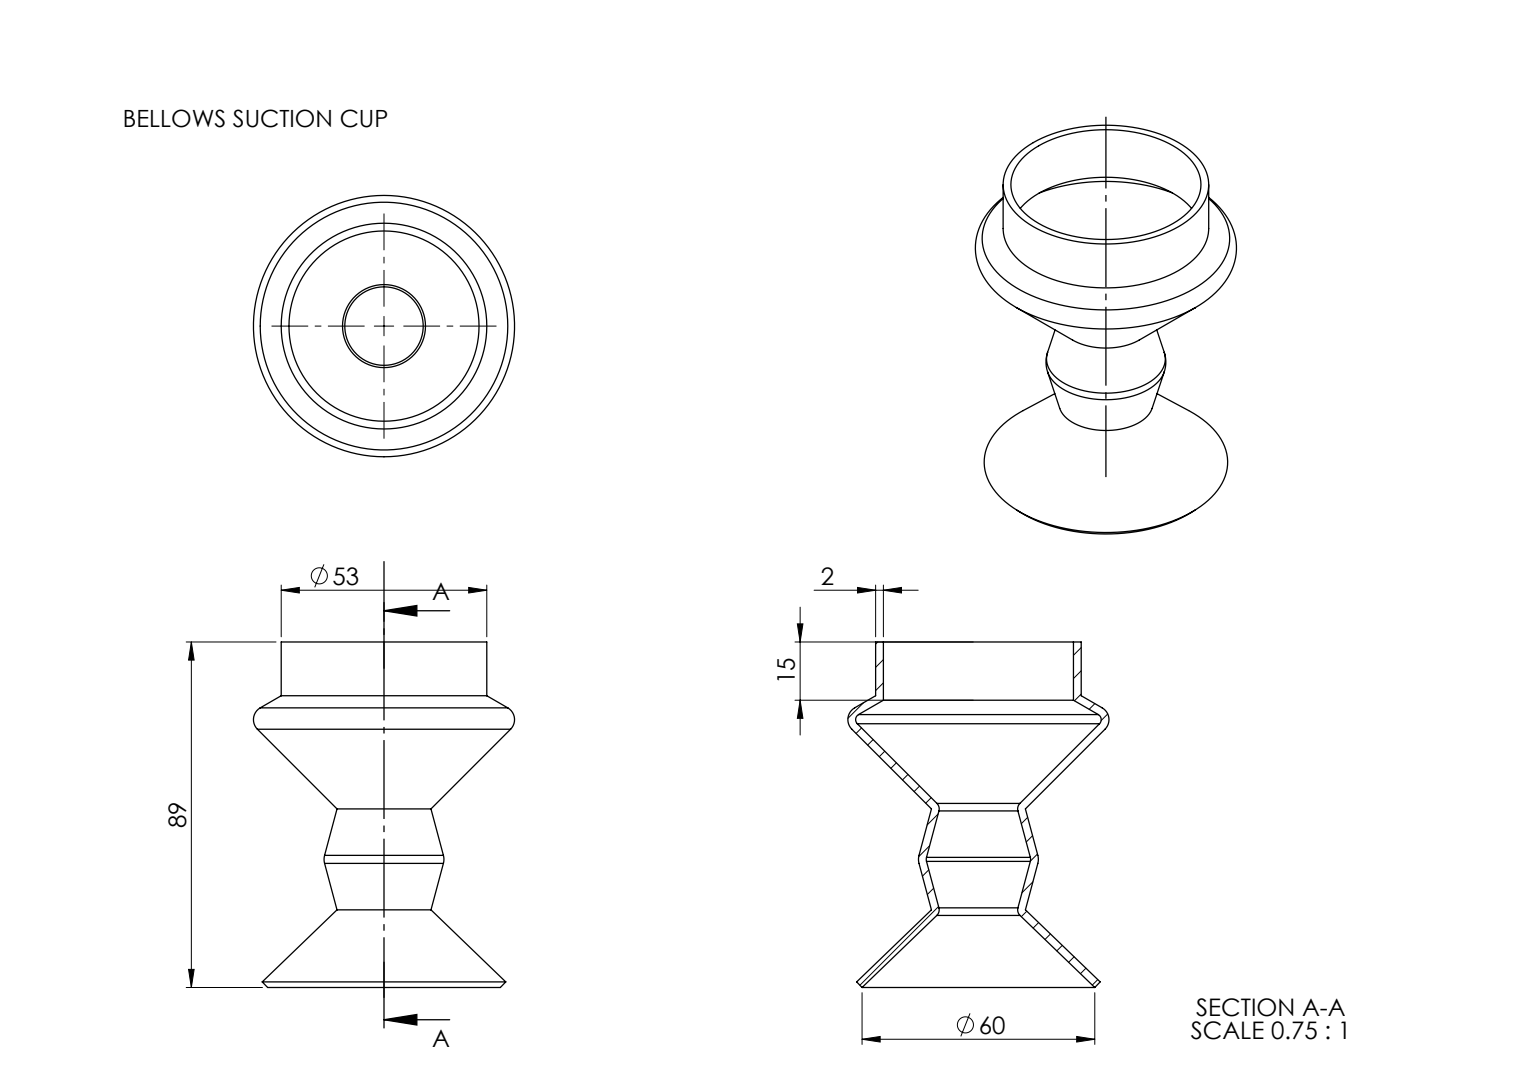
ISO-10303-21;
HEADER;
FILE_DESCRIPTION (('STEP AP214'),
    '1' );
FILE_NAME ('bellows suction cup.step',
    '2026-10-02T18:08:48',
    ( '' ),
    ( '' ),
    'SwSTEP 2.0',
    'SolidWorks 2026',
    '' );
FILE_SCHEMA (( 'AUTOMOTIVE_DESIGN' ));
ENDSEC;

DATA;
#110=CARTESIAN_POINT ( 'NONE',  ( 2.757615341152813402E-15, -45.51763809020504681, 0.000000000000000000 ) ) ;
#122=CARTESIAN_POINT ( 'NONE',  ( 0.000000000000000000, -21.99999999999999645, 0.000000000000000000 ) ) ;
#136=CIRCLE ( 'NONE', #19335, 15.31593959127081384 ) ;
#143=DIRECTION ( 'NONE',  ( -1.224646799147353454E-16, 1.000000000000000000, -0.000000000000000000 ) ) ;
#174=EDGE_LOOP ( 'NONE', ( #26748, #4103, #22808, #13833 ) ) ;
#178=CARTESIAN_POINT ( 'NONE',  ( 31.22091420962414787, -23.06066017177981209, 3.823459265327032686E-15 ) ) ;
#199=ORIENTED_EDGE ( 'NONE', *, *, #10938, .T. ) ;
#210=CLOSED_SHELL ( 'NONE', ( #8729, #14117, #31790, #11042, #12512, #8597, #17021, #15792, #28040, #1353, #2874, #26985, #12292, #25228, #17408, #25082, #11130, #24622, #12986, #14394, #9494, #16184, #21021, #7313, #8316, #7903, #7462, #29778, #24071, #10707, #8891, #2660, #1384, #1595, #31267, #2291, #15122, #887, #228, #13989, #650, #29273, #23959 ) ) ;
#213=CIRCLE ( 'NONE', #1854, 31.22091420962414787 ) ;
#215=DIRECTION ( 'NONE',  ( 1.224646799147353454E-16, -1.000000000000000000, 0.000000000000000000 ) ) ;
#228=ADVANCED_FACE ( 'NONE', ( #2232 ), #22152, .F. ) ;
#229=DIRECTION ( 'NONE',  ( 0.7202789989107551971, -0.6936844842780615084, 0.000000000000000000 ) ) ;
#231=( GEOMETRIC_REPRESENTATION_CONTEXT ( 3 ) GLOBAL_UNCERTAINTY_ASSIGNED_CONTEXT ( ( #25969 ) ) GLOBAL_UNIT_ASSIGNED_CONTEXT ( ( #31394, #13204, #25908 ) ) REPRESENTATION_CONTEXT ( 'NONE', 'WORKASPACE' ) );
#237=AXIS2_PLACEMENT_3D ( 'NONE', #10911, #18810, #13315 ) ;
#253=LINE ( 'NONE', #21716, #27788 ) ;
#265=DIRECTION ( 'NONE',  ( 1.224646799147353454E-16, -1.000000000000000000, 0.000000000000000000 ) ) ;
#266=ORIENTED_EDGE ( 'NONE', *, *, #7688, .T. ) ;
#281=FACE_OUTER_BOUND ( 'NONE', #10068, .T. ) ;
#284=DIRECTION ( 'NONE',  ( -1.224646799147353454E-16, 1.000000000000000000, -0.000000000000000000 ) ) ;
#374=CIRCLE ( 'NONE', #19015, 10.72870458603808075 ) ;
#401=CONICAL_SURFACE ( 'NONE', #22876, 24.50000000000000000, 0.7853981633974463916 ) ;
#429=CIRCLE ( 'NONE', #33304, 4.000000000000014211 ) ;
#464=DIRECTION ( 'NONE',  ( -1.000000000000000000, 0.000000000000000000, 0.000000000000000000 ) ) ;
#474=ORIENTED_EDGE ( 'NONE', *, *, #17841, .F. ) ;
#555=FACE_OUTER_BOUND ( 'NONE', #3316, .T. ) ;
#628=DIRECTION ( 'NONE',  ( -1.224646799147353454E-16, 1.000000000000000000, -0.000000000000000000 ) ) ;
#650=ADVANCED_FACE ( 'NONE', ( #26598 ), #1853, .T. ) ;
#676=AXIS2_PLACEMENT_3D ( 'NONE', #19715, #30162, #1674 ) ;
#706=CARTESIAN_POINT ( 'NONE',  ( 2.757615341152813402E-15, -45.51763809020504681, 0.000000000000000000 ) ) ;
#708=DIRECTION ( 'NONE',  ( 0.000000000000000000, -0.000000000000000000, -1.000000000000000000 ) ) ;
#869=APPLICATION_CONTEXT ( 'automotive_design' ) ;
#887=ADVANCED_FACE ( 'NONE', ( #25022 ), #29271, .F. ) ;
#958=DIRECTION ( 'NONE',  ( -1.000000000000000000, 0.000000000000000000, 0.000000000000000000 ) ) ;
#1000=DIRECTION ( 'NONE',  ( -1.224646799147353454E-16, 1.000000000000000000, -0.000000000000000000 ) ) ;
#1009=EDGE_LOOP ( 'NONE', ( #6385, #19811, #24661, #9041 ) ) ;
#1026=CARTESIAN_POINT ( 'NONE',  ( -8.761981113183991350E-16, -15.84529946162075298, 0.000000000000000000 ) ) ;
#1032=ORIENTED_EDGE ( 'NONE', *, *, #9068, .F. ) ;
#1054=ORIENTED_EDGE ( 'NONE', *, *, #1897, .T. ) ;
#1063=EDGE_CURVE ( 'NONE', #21883, #11212, #23262, .T. ) ;
#1088=VERTEX_POINT ( 'NONE', #12842 ) ;
#1136=AXIS2_PLACEMENT_3D ( 'NONE', #18668, #12050, #13680 ) ;
#1137=CIRCLE ( 'NONE', #17065, 10.11000150615022264 ) ;
#1163=DIRECTION ( 'NONE',  ( 0.2588190451025240146, -0.9659258262890673130, 0.000000000000000000 ) ) ;
#1165=FACE_OUTER_BOUND ( 'NONE', #17941, .T. ) ;
#1195=DIRECTION ( 'NONE',  ( -1.000000000000000000, 0.000000000000000000, 0.000000000000000000 ) ) ;
#1257=ORIENTED_EDGE ( 'NONE', *, *, #27744, .T. ) ;
#1353=ADVANCED_FACE ( 'NONE', ( #14831 ), #15022, .F. ) ;
#1355=DIRECTION ( 'NONE',  ( -1.000000000000000000, -1.309225264888156377E-16, 0.000000000000000000 ) ) ;
#1376=AXIS2_PLACEMENT_3D ( 'NONE', #6186, #27460, #21818 ) ;
#1384=ADVANCED_FACE ( 'NONE', ( #23749 ), #5887, .F. ) ;
#1388=VECTOR ( 'NONE', #20093, 999.9999999999998863 ) ;
#1443=DIRECTION ( 'NONE',  ( -1.224646799147353454E-16, 1.000000000000000000, -0.000000000000000000 ) ) ;
#1465=AXIS2_PLACEMENT_3D ( 'NONE', #20580, #4942, #2371 ) ;
#1503=DIRECTION ( 'NONE',  ( -1.224646799147353454E-16, 1.000000000000000000, -0.000000000000000000 ) ) ;
#1561=EDGE_LOOP ( 'NONE', ( #16202, #13374, #12638, #10013 ) ) ;
#1595=ADVANCED_FACE ( 'NONE', ( #555 ), #27605, .F. ) ;
#1608=DIRECTION ( 'NONE',  ( -1.224646799147353454E-16, 1.000000000000000000, -0.000000000000000000 ) ) ;
#1612=CARTESIAN_POINT ( 'NONE',  ( -10.11000150615021909, -45.00000000000000000, 0.000000000000000000 ) ) ;
#1674=DIRECTION ( 'NONE',  ( -1.000000000000000000, -1.416100796715761110E-16, 0.000000000000000000 ) ) ;
#1707=CIRCLE ( 'NONE', #20926, 10.18398033115917656 ) ;
#1766=CARTESIAN_POINT ( 'NONE',  ( 2.757615341152813402E-15, -45.51763809020504681, 0.000000000000000000 ) ) ;
#1770=AXIS2_PLACEMENT_3D ( 'NONE', #2717, #20916, #25712 ) ;
#1797=AXIS2_PLACEMENT_3D ( 'NONE', #2551, #23660, #26230 ) ;
#1853=TOROIDAL_SURFACE ( 'NONE', #7348, 12.11607355459420177, 2.000000000000000000 ) ;
#1854=AXIS2_PLACEMENT_3D ( 'NONE', #13967, #24431, #32646 ) ;
#1864=CARTESIAN_POINT ( 'NONE',  ( 13.38432950954957512, -58.51673569255127205, 1.639107629260334588E-15 ) ) ;
#1886=ORIENTED_EDGE ( 'NONE', *, *, #20671, .F. ) ;
#1897=EDGE_CURVE ( 'NONE', #21971, #4339, #29772, .T. ) ;
#1957=ORIENTED_EDGE ( 'NONE', *, *, #17449, .T. ) ;
#1981=FACE_OUTER_BOUND ( 'NONE', #8042, .T. ) ;
#1996=ORIENTED_EDGE ( 'NONE', *, *, #9547, .T. ) ;
#2013=TOROIDAL_SURFACE ( 'NONE', #21222, 12.11607355459420177, 2.000000000000000000 ) ;
#2034=DIRECTION ( 'NONE',  ( -1.224646799147353454E-16, 1.000000000000000000, -0.000000000000000000 ) ) ;
#2232=FACE_OUTER_BOUND ( 'NONE', #1009, .T. ) ;
#2254=VERTEX_POINT ( 'NONE', #178 ) ;
#2262=FACE_OUTER_BOUND ( 'NONE', #5128, .T. ) ;
#2265=TOROIDAL_SURFACE ( 'NONE', #29108, 12.11607355459420177, 2.000000000000000000 ) ;
#2291=ADVANCED_FACE ( 'NONE', ( #13746 ), #401, .F. ) ;
#2357=CIRCLE ( 'NONE', #6728, 12.11607355459420354 ) ;
#2367=FACE_OUTER_BOUND ( 'NONE', #33613, .T. ) ;
#2371=DIRECTION ( 'NONE',  ( -1.000000000000000000, 0.000000000000000000, 0.000000000000000000 ) ) ;
#2379=EDGE_CURVE ( 'NONE', #7355, #7743, #13581, .T. ) ;
#2383=AXIS2_PLACEMENT_3D ( 'NONE', #26930, #10991, #16152 ) ;
#2387=ORIENTED_EDGE ( 'NONE', *, *, #22718, .T. ) ;
#2402=SURFACE_SIDE_STYLE ('',( #5653 ) ) ;
#2408=AXIS2_PLACEMENT_3D ( 'NONE', #21011, #215, #25978 ) ;
#2453=DIRECTION ( 'NONE',  ( 0.2588190451025257355, -0.9659258262890668689, 0.000000000000000000 ) ) ;
#2480=COLOUR_RGB ( '', 0.66274510, 0.83137255, 0.94901961) ;
#2481=EDGE_LOOP ( 'NONE', ( #22705, #4855, #29179, #20689 ) ) ;
#2551=CARTESIAN_POINT ( 'NONE',  ( 2.694222958124179176E-15, -45.00000000000001421, 0.000000000000000000 ) ) ;
#2593=CARTESIAN_POINT ( 'NONE',  ( 11.45223628611453215, -57.99999999999999289, 1.402494451086933009E-15 ) ) ;
#2601=AXIS2_PLACEMENT_3D ( 'NONE', #3611, #27453, #1355 ) ;
#2660=ADVANCED_FACE ( 'NONE', ( #12691, #12522 ), #4281, .F. ) ;
#2690=ORIENTED_EDGE ( 'NONE', *, *, #25523, .T. ) ;
#2717=CARTESIAN_POINT ( 'NONE',  ( -2.815509657234710744E-16, -20.70096189432334555, 0.000000000000000000 ) ) ;
#2720=FACE_OUTER_BOUND ( 'NONE', #7788, .T. ) ;
#2729=EDGE_LOOP ( 'NONE', ( #11660, #5888, #17586, #12988 ) ) ;
#2789=CARTESIAN_POINT ( 'NONE',  ( 30.00000000000001066, -91.00000000000000000, 0.000000000000000000 ) ) ;
#2856=CARTESIAN_POINT ( 'NONE',  ( 24.50000000000000000, -16.99999999999999289, 3.000384657911015469E-15 ) ) ;
#2874=ADVANCED_FACE ( 'NONE', ( #5478 ), #31637, .T. ) ;
#2898=ORIENTED_EDGE ( 'NONE', *, *, #20671, .T. ) ;
#2940=EDGE_LOOP ( 'NONE', ( #4959, #14793, #18981, #27682 ) ) ;
#2949=DIRECTION ( 'NONE',  ( 0.000000000000000000, -0.000000000000000000, -1.000000000000000000 ) ) ;
#3047=DIRECTION ( 'NONE',  ( -0.7071067811865462405, 0.7071067811865489050, 0.000000000000000000 ) ) ;
#3083=CARTESIAN_POINT ( 'NONE',  ( 5.204170427930421283E-15, -70.99969134886156041, 0.000000000000000000 ) ) ;
#3143=AXIS2_PLACEMENT_3D ( 'NONE', #16484, #26940, #3440 ) ;
#3150=DIRECTION ( 'NONE',  ( -1.000000000000000000, -1.416100796715761110E-16, 0.000000000000000000 ) ) ;
#3165=AXIS2_PLACEMENT_3D ( 'NONE', #16128, #3242, #24176 ) ;
#3191=AXIS2_PLACEMENT_3D ( 'NONE', #22795, #4600, #25545 ) ;
#3242=DIRECTION ( 'NONE',  ( -1.224646799147353454E-16, 1.000000000000000000, -0.000000000000000000 ) ) ;
#3289=EDGE_CURVE ( 'NONE', #15868, #29257, #7629, .T. ) ;
#3316=EDGE_LOOP ( 'NONE', ( #474, #19189, #20666, #19232 ) ) ;
#3375=VECTOR ( 'NONE', #16248, 1000.000000000000114 ) ;
#3422=EDGE_CURVE ( 'NONE', #4339, #20029, #29557, .T. ) ;
#3440=DIRECTION ( 'NONE',  ( 1.000000000000000000, 0.000000000000000000, 1.224646799147352714E-16 ) ) ;
#3450=DIRECTION ( 'NONE',  ( 1.224646799147353454E-16, -1.000000000000000000, 0.000000000000000000 ) ) ;
#3455=AXIS2_PLACEMENT_3D ( 'NONE', #29112, #7846, #8183 ) ;
#3465=DIRECTION ( 'NONE',  ( -1.000000000000000000, 0.000000000000000000, 0.000000000000000000 ) ) ;
#3487=ORIENTED_EDGE ( 'NONE', *, *, #23060, .T. ) ;
#3554=LINE ( 'NONE', #11609, #25895 ) ;
#3565=ORIENTED_EDGE ( 'NONE', *, *, #25296, .F. ) ;
#3608=AXIS2_PLACEMENT_3D ( 'NONE', #1026, #24229, #21987 ) ;
#3611=CARTESIAN_POINT ( 'NONE',  ( -8.761981113183991350E-16, -15.84529946162075298, 0.000000000000000000 ) ) ;
#3664=DIRECTION ( 'NONE',  ( 1.000000000000000000, 0.000000000000000000, 1.224646799147353947E-16 ) ) ;
#3707=EDGE_CURVE ( 'NONE', #11212, #14916, #27280, .T. ) ;
#3757=EDGE_CURVE ( 'NONE', #16950, #4399, #21280, .T. ) ;
#3768=DIRECTION ( 'NONE',  ( -0.2588190451025255689, -0.9659258262890669799, 3.169619151431825338E-17 ) ) ;
#3773=CARTESIAN_POINT ( 'NONE',  ( 3.469446951953614189E-15, -45.00000000000000000, 0.000000000000000000 ) ) ;
#3890=FILL_AREA_STYLE_COLOUR ( '', #2480 ) ;
#3963=CARTESIAN_POINT ( 'NONE',  ( 4.412827539393359662E-15, -59.03347138510255832, 0.000000000000000000 ) ) ;
#3970=AXIS2_PLACEMENT_3D ( 'NONE', #27710, #1443, #17589 ) ;
#3977=VERTEX_POINT ( 'NONE', #10259 ) ;
#4088=DIRECTION ( 'NONE',  ( 1.000000000000000000, 0.000000000000000000, 0.000000000000000000 ) ) ;
#4103=ORIENTED_EDGE ( 'NONE', *, *, #8318, .T. ) ;
#4130=ORIENTED_EDGE ( 'NONE', *, *, #27703, .T. ) ;
#4144=VECTOR ( 'NONE', #9708, 1000.000000000000114 ) ;
#4169=DIRECTION ( 'NONE',  ( -0.2588190451025238481, -0.9659258262890674240, 3.169619151431803768E-17 ) ) ;
#4196=FACE_OUTER_BOUND ( 'NONE', #4510, .T. ) ;
#4221=DIRECTION ( 'NONE',  ( -1.224646799147353454E-16, 1.000000000000000000, -0.000000000000000000 ) ) ;
#4244=CARTESIAN_POINT ( 'NONE',  ( 6.054684311146244891E-15, -72.44024934668307480, 0.000000000000000000 ) ) ;
#4276=ORIENTED_EDGE ( 'NONE', *, *, #9547, .F. ) ;
#4281=PLANE ( 'NONE',  #6435 ) ;
#4315=ORIENTED_EDGE ( 'NONE', *, *, #7894, .F. ) ;
#4339=VERTEX_POINT ( 'NONE', #20056 ) ;
#4356=ORIENTED_EDGE ( 'NONE', *, *, #7565, .T. ) ;
#4373=DIRECTION ( 'NONE',  ( -1.000000000000000000, 0.000000000000000000, 0.000000000000000000 ) ) ;
#4386=APPLICATION_CONTEXT ( 'automotive_design' ) ;
#4399=VERTEX_POINT ( 'NONE', #27772 ) ;
#4418=EDGE_CURVE ( 'NONE', #7411, #6369, #6462, .T. ) ;
#4430=LINE ( 'NONE', #17313, #13313 ) ;
#4507=CARTESIAN_POINT ( 'NONE',  ( -13.38432950954956624, -58.51673569255127205, 0.000000000000000000 ) ) ;
#4508=CARTESIAN_POINT ( 'NONE',  ( 15.31642273298461632, -59.03347138510255832, 1.875720807433735970E-15 ) ) ;
#4510=EDGE_LOOP ( 'NONE', ( #15697, #18450, #22380, #31090 ) ) ;
#4526=EDGE_CURVE ( 'NONE', #11830, #7617, #7016, .T. ) ;
#4531=CIRCLE ( 'NONE', #1770, 30.91025403784432868 ) ;
#4534=ORIENTED_EDGE ( 'NONE', *, *, #1063, .T. ) ;
#4536=CIRCLE ( 'NONE', #10037, 24.49999999999999645 ) ;
#4539=CARTESIAN_POINT ( 'NONE',  ( 2.521031746877078694E-15, -43.58578643762690064, 0.000000000000000000 ) ) ;
#4600=DIRECTION ( 'NONE',  ( -1.224646799147353454E-16, 1.000000000000000000, -0.000000000000000000 ) ) ;
#4602=DIRECTION ( 'NONE',  ( -1.000000000000000000, 0.000000000000000000, 0.000000000000000000 ) ) ;
#4609=EDGE_CURVE ( 'NONE', #7355, #27495, #33250, .T. ) ;
#4623=CARTESIAN_POINT ( 'NONE',  ( -26.50000000000000355, -2.000000000000000000, 0.000000000000000000 ) ) ;
#4635=CARTESIAN_POINT ( 'NONE',  ( 32.63512777199724724, -24.47487373415290790, 3.996650476574133167E-15 ) ) ;
#4665=ORIENTED_EDGE ( 'NONE', *, *, #3422, .T. ) ;
#4679=DIRECTION ( 'NONE',  ( -1.000000000000000000, -1.224646799147353454E-16, 0.000000000000000000 ) ) ;
#4682=ORIENTED_EDGE ( 'NONE', *, *, #29841, .T. ) ;
#4708=CARTESIAN_POINT ( 'NONE',  ( 7.428728520588063561E-18, -23.06066017177981564, 0.000000000000000000 ) ) ;
#4855=ORIENTED_EDGE ( 'NONE', *, *, #12029, .T. ) ;
#4915=ORIENTED_EDGE ( 'NONE', *, *, #8318, .F. ) ;
#4931=SHAPE_DEFINITION_REPRESENTATION ( #13749, #19696 ) ;
#4942=DIRECTION ( 'NONE',  ( -1.224646799147353454E-16, 1.000000000000000000, -0.000000000000000000 ) ) ;
#4952=PRODUCT ( 'bellows suction cup', 'bellows suction cup', '', ( #23473 ) ) ;
#4959=ORIENTED_EDGE ( 'NONE', *, *, #27703, .F. ) ;
#5000=ORIENTED_EDGE ( 'NONE', *, *, #11667, .F. ) ;
#5007=DIRECTION ( 'NONE',  ( -1.224646799147353207E-16, -1.499759782661857882E-32, 1.000000000000000000 ) ) ;
#5021=FACE_OUTER_BOUND ( 'NONE', #24340, .T. ) ;
#5042=EDGE_CURVE ( 'NONE', #28529, #17976, #11406, .T. ) ;
#5044=CARTESIAN_POINT ( 'NONE',  ( -29.99999999999999645, -91.00000000000000000, 3.673940397442059967E-15 ) ) ;
#5128=EDGE_LOOP ( 'NONE', ( #30565, #20332, #24416, #11247 ) ) ;
#5131=ORIENTED_EDGE ( 'NONE', *, *, #16178, .T. ) ;
#5143=PRESENTATION_STYLE_ASSIGNMENT (( #12870 ) ) ;
#5178=EDGE_CURVE ( 'NONE', #6369, #7411, #5928, .T. ) ;
#5187=DIRECTION ( 'NONE',  ( -0.8660254037844369313, -0.5000000000000028866, 1.060575238724904943E-16 ) ) ;
#5201=AXIS2_PLACEMENT_3D ( 'NONE', #9756, #9587, #15086 ) ;
#5259=EDGE_LOOP ( 'NONE', ( #28388, #30221, #18020, #27449 ) ) ;
#5271=DIRECTION ( 'NONE',  ( -1.224646799147353454E-16, 1.000000000000000000, -0.000000000000000000 ) ) ;
#5285=DIRECTION ( 'NONE',  ( -0.6936844842780661713, 0.7202789989107508672, 0.000000000000000000 ) ) ;
#5286=EDGE_CURVE ( 'NONE', #20029, #1088, #429, .T. ) ;
#5312=DIRECTION ( 'NONE',  ( 0.2583678462756400229, 0.9660466117175129375, 3.164093559440580996E-17 ) ) ;
#5385=VERTEX_POINT ( 'NONE', #27561 ) ;
#5430=CARTESIAN_POINT ( 'NONE',  ( 3.469446951953614189E-15, -45.00000000000000000, 0.000000000000000000 ) ) ;
#5478=FACE_OUTER_BOUND ( 'NONE', #19566, .T. ) ;
#5559=ORIENTED_EDGE ( 'NONE', *, *, #9068, .T. ) ;
#5582=CIRCLE ( 'NONE', #9960, 26.50000000000000000 ) ;
#5597=ORIENTED_EDGE ( 'NONE', *, *, #11873, .T. ) ;
#5600=EDGE_CURVE ( 'NONE', #7743, #23590, #21725, .T. ) ;
#5645=ORIENTED_EDGE ( 'NONE', *, *, #12029, .F. ) ;
#5653=SURFACE_STYLE_FILL_AREA ( #29319 ) ;
#5672=AXIS2_PLACEMENT_3D ( 'NONE', #23110, #23461, #33923 ) ;
#5817=CIRCLE ( 'NONE', #7458, 10.17814985357208890 ) ;
#5830=CARTESIAN_POINT ( 'NONE',  ( 5.204170427930421283E-15, -70.99969134886156041, 0.000000000000000000 ) ) ;
#5838=DIRECTION ( 'NONE',  ( -0.7202789989107549751, -0.6936844842780617304, 8.820873705091161919E-17 ) ) ;
#5887=CYLINDRICAL_SURFACE ( 'NONE', #33662, 24.49999999999999645 ) ;
#5888=ORIENTED_EDGE ( 'NONE', *, *, #24657, .F. ) ;
#5900=EDGE_CURVE ( 'NONE', #1088, #9464, #33248, .T. ) ;
#5928=CIRCLE ( 'NONE', #25094, 13.38432950954957157 ) ;
#6007=ORIENTED_EDGE ( 'NONE', *, *, #23213, .T. ) ;
#6141=DIRECTION ( 'NONE',  ( 1.224646799147353454E-16, -1.000000000000000000, 0.000000000000000000 ) ) ;
#6169=AXIS2_PLACEMENT_3D ( 'NONE', #11647, #32574, #17149 ) ;
#6186=CARTESIAN_POINT ( 'NONE',  ( 0.000000000000000000, 0.000000000000000000, 0.000000000000000000 ) ) ;
#6190=AXIS2_PLACEMENT_3D ( 'NONE', #32901, #9400, #19883 ) ;
#6220=AXIS2_PLACEMENT_3D ( 'NONE', #24367, #19056, #14067 ) ;
#6224=VERTEX_POINT ( 'NONE', #5044 ) ;
#6245=AXIS2_PLACEMENT_3D ( 'NONE', #6662, #25544, #4088 ) ;
#6275=EDGE_CURVE ( 'NONE', #29257, #31380, #12941, .T. ) ;
#6312=MECHANICAL_DESIGN_GEOMETRIC_PRESENTATION_REPRESENTATION('',(#28758),#28244);
#6336=CARTESIAN_POINT ( 'NONE',  ( 10.18398033115918189, -70.48295565631028126, 1.443142760386851780E-15 ) ) ;
#6346=CARTESIAN_POINT ( 'NONE',  ( -10.11607355459419644, -70.99969134886156041, 0.000000000000000000 ) ) ;
#6369=VERTEX_POINT ( 'NONE', #18613 ) ;
#6380=EDGE_CURVE ( 'NONE', #7743, #14916, #15865, .T. ) ;
#6385=ORIENTED_EDGE ( 'NONE', *, *, #30392, .F. ) ;
#6393=CARTESIAN_POINT ( 'NONE',  ( 24.49999999999999645, -22.99999999999999645, 3.000384657911015074E-15 ) ) ;
#6398=CIRCLE ( 'NONE', #1465, 30.00000000000000711 ) ;
#6407=DIRECTION ( 'NONE',  ( -1.224646799147353207E-16, -1.499759782661857882E-32, 1.000000000000000000 ) ) ;
#6409=VECTOR ( 'NONE', #31627, 1000.000000000000000 ) ;
#6435=AXIS2_PLACEMENT_3D ( 'NONE', #4623, #25733, #12862 ) ;
#6437=DIRECTION ( 'NONE',  ( -1.000000000000000000, -1.224646799147353454E-16, 0.000000000000000000 ) ) ;
#6462=CIRCLE ( 'NONE', #9190, 13.38432950954957157 ) ;
#6574=CARTESIAN_POINT ( 'NONE',  ( -7.347880794884122694E-16, -16.99999999999999645, 0.000000000000000000 ) ) ;
#6593=CARTESIAN_POINT ( 'NONE',  ( 4.159479030958464888E-15, -56.96472381958990638, 0.000000000000000000 ) ) ;
#6600=EDGE_LOOP ( 'NONE', ( #30266, #4130, #15362, #12431 ) ) ;
#6662=CARTESIAN_POINT ( 'NONE',  ( 2.757615341152813402E-15, -45.51763809020504681, 0.000000000000000000 ) ) ;
#6696=FACE_OUTER_BOUND ( 'NONE', #2729, .T. ) ;
#6701=ORIENTED_EDGE ( 'NONE', *, *, #5600, .F. ) ;
#6724=LINE ( 'NONE', #6393, #23733 ) ;
#6728=AXIS2_PLACEMENT_3D ( 'NONE', #22944, #25686, #7146 ) ;
#6756=AXIS2_PLACEMENT_3D ( 'NONE', #122, #10614, #20758 ) ;
#6780=AXIS2_PLACEMENT_3D ( 'NONE', #33203, #30630, #9706 ) ;
#6845=EDGE_CURVE ( 'NONE', #28463, #33921, #21228, .T. ) ;
#6849=CARTESIAN_POINT ( 'NONE',  ( 24.49999999999999289, -1.999999999999995337, 3.000384657911015074E-15 ) ) ;
#6866=LINE ( 'NONE', #30885, #1388 ) ;
#6869=ORIENTED_EDGE ( 'NONE', *, *, #32222, .T. ) ;
#6905=VECTOR ( 'NONE', #3047, 999.9999999999998863 ) ;
#6909=CARTESIAN_POINT ( 'NONE',  ( -10.17814985357208535, -45.51763809020504681, 1.246463863941915894E-15 ) ) ;
#6976=VERTEX_POINT ( 'NONE', #6346 ) ;
#7016=CIRCLE ( 'NONE', #3191, 24.49999999999999645 ) ;
#7146=DIRECTION ( 'NONE',  ( -1.000000000000000000, 0.000000000000000000, 0.000000000000000000 ) ) ;
#7258=EDGE_CURVE ( 'NONE', #25648, #9464, #13557, .T. ) ;
#7279=DIRECTION ( 'NONE',  ( -1.000000000000000000, -1.111257322145974683E-16, 0.000000000000000000 ) ) ;
#7289=CYLINDRICAL_SURFACE ( 'NONE', #27068, 26.50000000000000000 ) ;
#7313=ADVANCED_FACE ( 'NONE', ( #20595 ), #22849, .T. ) ;
#7348=AXIS2_PLACEMENT_3D ( 'NONE', #5830, #16309, #26765 ) ;
#7355=VERTEX_POINT ( 'NONE', #27790 ) ;
#7381=FACE_OUTER_BOUND ( 'NONE', #10798, .T. ) ;
#7411=VERTEX_POINT ( 'NONE', #1864 ) ;
#7457=VERTEX_POINT ( 'NONE', #2856 ) ;
#7458=AXIS2_PLACEMENT_3D ( 'NONE', #706, #11192, #20998 ) ;
#7462=ADVANCED_FACE ( 'NONE', ( #22811 ), #20355, .T. ) ;
#7519=AXIS2_PLACEMENT_3D ( 'NONE', #3773, #19565, #27281 ) ;
#7533=EDGE_LOOP ( 'NONE', ( #12921, #21559, #5131, #12948 ) ) ;
#7565=EDGE_CURVE ( 'NONE', #33921, #28463, #1137, .T. ) ;
#7581=TOROIDAL_SURFACE ( 'NONE', #28853, 30.16025403784430736, 3.500000000000010658 ) ;
#7617=VERTEX_POINT ( 'NONE', #6849 ) ;
#7629=LINE ( 'NONE', #8297, #24513 ) ;
#7677=CARTESIAN_POINT ( 'NONE',  ( 6.054684311146244891E-15, -72.44024934668307480, 0.000000000000000000 ) ) ;
#7680=DIRECTION ( 'NONE',  ( -1.000000000000000000, 0.000000000000000000, 0.000000000000000000 ) ) ;
#7688=EDGE_CURVE ( 'NONE', #23106, #2254, #12165, .T. ) ;
#7689=FACE_OUTER_BOUND ( 'NONE', #32083, .T. ) ;
#7743=VERTEX_POINT ( 'NONE', #24459 ) ;
#7751=DIRECTION ( 'NONE',  ( -1.000000000000000000, -1.224646799147353454E-16, 0.000000000000000000 ) ) ;
#7752=AXIS2_PLACEMENT_3D ( 'NONE', #17729, #25954, #33327 ) ;
#7780=AXIS2_PLACEMENT_3D ( 'NONE', #25350, #12307, #15584 ) ;
#7788=EDGE_LOOP ( 'NONE', ( #3565, #9159, #26412, #199 ) ) ;
#7822=CIRCLE ( 'NONE', #16072, 31.22091420962414787 ) ;
#7838=TOROIDAL_SURFACE ( 'NONE', #27017, 12.11000150615021553, 1.999999999999992228 ) ;
#7846=DIRECTION ( 'NONE',  ( -1.224646799147353454E-16, 1.000000000000000000, -0.000000000000000000 ) ) ;
#7849=DIRECTION ( 'NONE',  ( -1.000000000000000000, 0.000000000000000000, 0.000000000000000000 ) ) ;
#7857=CARTESIAN_POINT ( 'NONE',  ( -31.22091420962414787, -23.06066017177981919, 0.000000000000000000 ) ) ;
#7894=EDGE_CURVE ( 'NONE', #18620, #6224, #31838, .T. ) ;
#7903=ADVANCED_FACE ( 'NONE', ( #4196 ), #14881, .T. ) ;
#7922=CARTESIAN_POINT ( 'NONE',  ( 12.11000150615021909, -45.00000000000000000, 1.483047458217648827E-15 ) ) ;
#7935=CARTESIAN_POINT ( 'NONE',  ( 0.000000000000000000, -21.99999999999999645, 0.000000000000000000 ) ) ;
#7998=AXIS2_PLACEMENT_3D ( 'NONE', #32435, #29863, #16842 ) ;
#8001=ORIENTED_EDGE ( 'NONE', *, *, #22244, .F. ) ;
#8021=CARTESIAN_POINT ( 'NONE',  ( 5.814984965855610735E-15, -70.48295565631028126, 0.000000000000000000 ) ) ;
#8042=EDGE_LOOP ( 'NONE', ( #4534, #24009, #8001, #1886 ) ) ;
#8079=AXIS2_PLACEMENT_3D ( 'NONE', #16861, #27321, #20637 ) ;
#8131=VECTOR ( 'NONE', #23794, 1000.000000000000000 ) ;
#8156=DIRECTION ( 'NONE',  ( 0.2583678462756386907, 0.9660466117175132705, 3.164093559440564356E-17 ) ) ;
#8183=DIRECTION ( 'NONE',  ( -1.000000000000000000, -1.087251435804610394E-16, 0.000000000000000000 ) ) ;
#8195=DIRECTION ( 'NONE',  ( -1.224646799147353454E-16, 1.000000000000000000, -0.000000000000000000 ) ) ;
#8255=PRODUCT_DEFINITION ( 'UNKNOWN', '', #14809, #19552 ) ;
#8286=CONICAL_SURFACE ( 'NONE', #25293, 10.72870458603808075, 0.8042044335707554392 ) ;
#8297=CARTESIAN_POINT ( 'NONE',  ( 10.72870458603808608, -72.44024934668307480, 0.000000000000000000 ) ) ;
#8316=ADVANCED_FACE ( 'NONE', ( #18370 ), #12678, .T. ) ;
#8318=EDGE_CURVE ( 'NONE', #29257, #6224, #20927, .T. ) ;
#8324=EDGE_CURVE ( 'NONE', #21971, #25648, #20608, .T. ) ;
#8358=CARTESIAN_POINT ( 'NONE',  ( 4.222871413987100692E-15, -57.48236190979495319, 0.000000000000000000 ) ) ;
#8370=ORIENTED_EDGE ( 'NONE', *, *, #14830, .T. ) ;
#8372=ORIENTED_EDGE ( 'NONE', *, *, #11319, .F. ) ;
#8597=ADVANCED_FACE ( 'NONE', ( #26587 ), #8286, .F. ) ;
#8631=DIRECTION ( 'NONE',  ( -1.000000000000000000, 0.000000000000000000, 0.000000000000000000 ) ) ;
#8682=DIRECTION ( 'NONE',  ( -1.000000000000000000, -1.063101997391471025E-16, 0.000000000000000000 ) ) ;
#8729=ADVANCED_FACE ( 'NONE', ( #16626 ), #2265, .T. ) ;
#8737=CARTESIAN_POINT ( 'NONE',  ( -10.17814985357208535, -45.51763809020504681, 0.000000000000000000 ) ) ;
#8845=CIRCLE ( 'NONE', #25292, 10.11607355459420177 ) ;
#8891=ADVANCED_FACE ( 'NONE', ( #11797 ), #27418, .T. ) ;
#8908=CONICAL_SURFACE ( 'NONE', #33581, 30.00000000000000711, 0.7665918932241471140 ) ;
#8911=CIRCLE ( 'NONE', #13317, 1.999999999999993117 ) ;
#8938=CONICAL_SURFACE ( 'NONE', #17725, 32.63512777199724724, 0.7853981633974471688 ) ;
#8990=CARTESIAN_POINT ( 'NONE',  ( 32.63512777199724724, -24.47487373415290790, 3.996650476574133167E-15 ) ) ;
#9041=ORIENTED_EDGE ( 'NONE', *, *, #30437, .T. ) ;
#9068=EDGE_CURVE ( 'NONE', #12231, #28463, #11073, .T. ) ;
#9071=DIRECTION ( 'NONE',  ( -1.224646799147353454E-16, 1.000000000000000000, -0.000000000000000000 ) ) ;
#9080=EDGE_CURVE ( 'NONE', #23590, #27495, #5582, .T. ) ;
#9086=CIRCLE ( 'NONE', #28279, 2.000000000000013767 ) ;
#9124=ORIENTED_EDGE ( 'NONE', *, *, #27744, .F. ) ;
#9159=ORIENTED_EDGE ( 'NONE', *, *, #27274, .F. ) ;
#9190=AXIS2_PLACEMENT_3D ( 'NONE', #30500, #25023, #27431 ) ;
#9344=DIRECTION ( 'NONE',  ( -1.224646799147353454E-16, 1.000000000000000000, -0.000000000000000000 ) ) ;
#9372=CIRCLE ( 'NONE', #25834, 31.38736896855613523 ) ;
#9400=DIRECTION ( 'NONE',  ( -1.224646799147353454E-16, 1.000000000000000000, -0.000000000000000000 ) ) ;
#9441=CONICAL_SURFACE ( 'NONE', #6169, 13.38432950954957157, 0.2613323016132363952 ) ;
#9464=VERTEX_POINT ( 'NONE', #28228 ) ;
#9466=DIRECTION ( 'NONE',  ( -1.000000000000000000, 0.000000000000000000, 0.000000000000000000 ) ) ;
#9483=ORIENTED_EDGE ( 'NONE', *, *, #5286, .F. ) ;
#9494=ADVANCED_FACE ( 'NONE', ( #25994 ), #25855, .T. ) ;
#9523=FACE_OUTER_BOUND ( 'NONE', #26108, .T. ) ;
#9540=STYLED_ITEM ( 'NONE', ( #5143 ), #15260 ) ;
#9547=EDGE_CURVE ( 'NONE', #12231, #23106, #14342, .T. ) ;
#9587=DIRECTION ( 'NONE',  ( -1.224646799147353454E-16, 1.000000000000000000, -0.000000000000000000 ) ) ;
#9593=AXIS2_PLACEMENT_3D ( 'NONE', #17629, #20555, #28090 ) ;
#9594=DIRECTION ( 'NONE',  ( 0.7071067811865460184, 0.7071067811865489050, 8.659560562354914369E-17 ) ) ;
#9643=DIRECTION ( 'NONE',  ( -1.000000000000000000, -1.239088197126291063E-16, 0.000000000000000000 ) ) ;
#9706=DIRECTION ( 'NONE',  ( -1.000000000000000000, -1.309225264888156377E-16, 0.000000000000000000 ) ) ;
#9708=DIRECTION ( 'NONE',  ( 0.7202789989107551971, -0.6936844842780615084, 0.000000000000000000 ) ) ;
#9756=CARTESIAN_POINT ( 'NONE',  ( -2.571758278209442450E-15, -1.999999999999998224, 0.000000000000000000 ) ) ;
#9829=DIRECTION ( 'NONE',  ( -0.2583678462756388572, 0.9660466117175131595, 0.000000000000000000 ) ) ;
#9865=DIRECTION ( 'NONE',  ( -1.000000000000000000, -1.224646799147353454E-16, 0.000000000000000000 ) ) ;
#9960=AXIS2_PLACEMENT_3D ( 'NONE', #12482, #5271, #17988 ) ;
#10013=ORIENTED_EDGE ( 'NONE', *, *, #13215, .T. ) ;
#10035=ORIENTED_EDGE ( 'NONE', *, *, #32348, .T. ) ;
#10037=AXIS2_PLACEMENT_3D ( 'NONE', #26116, #18239, #20294 ) ;
#10068=EDGE_LOOP ( 'NONE', ( #18616, #17669, #31630, #5559 ) ) ;
#10093=DIRECTION ( 'NONE',  ( -1.224646799147353454E-16, 1.000000000000000000, -0.000000000000000000 ) ) ;
#10117=ORIENTED_EDGE ( 'NONE', *, *, #11873, .F. ) ;
#10135=DIRECTION ( 'NONE',  ( -1.224646799147353454E-16, 1.000000000000000000, -0.000000000000000000 ) ) ;
#10212=VECTOR ( 'NONE', #9829, 1000.000000000000114 ) ;
#10259=CARTESIAN_POINT ( 'NONE',  ( 10.11607355459420710, -70.99969134886156041, 1.238861709857297692E-15 ) ) ;
#10291=ORIENTED_EDGE ( 'NONE', *, *, #33593, .T. ) ;
#10316=DIRECTION ( 'NONE',  ( 1.000000000000000000, 0.000000000000000000, 1.224646799147353700E-16 ) ) ;
#10340=CARTESIAN_POINT ( 'NONE',  ( -30.16025403784430736, -22.00000000000000000, 0.000000000000000000 ) ) ;
#10372=ORIENTED_EDGE ( 'NONE', *, *, #22463, .T. ) ;
#10411=EDGE_LOOP ( 'NONE', ( #23839, #23627, #18896, #13145 ) ) ;
#10431=DIRECTION ( 'NONE',  ( -1.224646799147353454E-16, 1.000000000000000000, -0.000000000000000000 ) ) ;
#10573=CIRCLE ( 'NONE', #33001, 2.000000000000000000 ) ;
#10583=ORIENTED_EDGE ( 'NONE', *, *, #25296, .T. ) ;
#10601=CARTESIAN_POINT ( 'NONE',  ( -24.49999999999999645, -17.00000000000000000, 0.000000000000000000 ) ) ;
#10607=DIRECTION ( 'NONE',  ( -1.224646799147353454E-16, 1.000000000000000000, -0.000000000000000000 ) ) ;
#10614=DIRECTION ( 'NONE',  ( -1.224646799147353454E-16, 1.000000000000000000, -0.000000000000000000 ) ) ;
#10625=EDGE_LOOP ( 'NONE', ( #24914, #32419, #20889, #18532 ) ) ;
#10644=CONICAL_SURFACE ( 'NONE', #22685, 24.49999999999999645, 1.047197551196593412 ) ;
#10664=ORIENTED_EDGE ( 'NONE', *, *, #5900, .T. ) ;
#10683=CARTESIAN_POINT ( 'NONE',  ( 12.11000150615022264, -45.00000000000001421, 0.000000000000000000 ) ) ;
#10707=ADVANCED_FACE ( 'NONE', ( #6696 ), #15686, .T. ) ;
#10712=ORIENTED_EDGE ( 'NONE', *, *, #12161, .T. ) ;
#10772=DIRECTION ( 'NONE',  ( -1.000000000000000000, 0.000000000000000000, 0.000000000000000000 ) ) ;
#10798=EDGE_LOOP ( 'NONE', ( #23034, #23287, #13026, #15178 ) ) ;
#10803=DIRECTION ( 'NONE',  ( -1.224646799147353454E-16, 1.000000000000000000, -0.000000000000000000 ) ) ;
#10911=CARTESIAN_POINT ( 'NONE',  ( 3.469446951953614189E-15, -45.00000000000000000, 0.000000000000000000 ) ) ;
#10934=DIRECTION ( 'NONE',  ( -1.000000000000000000, -1.224646799147353454E-16, 0.000000000000000000 ) ) ;
#10938=EDGE_CURVE ( 'NONE', #4399, #20157, #28813, .T. ) ;
#10983=EDGE_CURVE ( 'NONE', #6369, #17976, #9086, .T. ) ;
#10991=DIRECTION ( 'NONE',  ( -1.224646799147353454E-16, 1.000000000000000000, -0.000000000000000000 ) ) ;
#11042=ADVANCED_FACE ( 'NONE', ( #7381 ), #22228, .T. ) ;
#11044=ORIENTED_EDGE ( 'NONE', *, *, #11319, .T. ) ;
#11073=CIRCLE ( 'NONE', #7780, 1.999999999999993117 ) ;
#11083=EDGE_LOOP ( 'NONE', ( #4315, #12754, #11455, #31462 ) ) ;
#11130=ADVANCED_FACE ( 'NONE', ( #20617 ), #17884, .T. ) ;
#11170=ORIENTED_EDGE ( 'NONE', *, *, #5900, .F. ) ;
#11192=DIRECTION ( 'NONE',  ( -1.224646799147353454E-16, 1.000000000000000000, -0.000000000000000000 ) ) ;
#11194=DIRECTION ( 'NONE',  ( -1.224646799147353454E-16, 1.000000000000000000, -0.000000000000000000 ) ) ;
#11212=VERTEX_POINT ( 'NONE', #4635 ) ;
#11247=ORIENTED_EDGE ( 'NONE', *, *, #10983, .F. ) ;
#11280=DIRECTION ( 'NONE',  ( -1.224646799147353454E-16, 1.000000000000000000, -0.000000000000000000 ) ) ;
#11291=EDGE_LOOP ( 'NONE', ( #31422, #6869, #10664, #23421 ) ) ;
#11293=ORIENTED_EDGE ( 'NONE', *, *, #3422, .F. ) ;
#11319=EDGE_CURVE ( 'NONE', #27878, #21883, #6866, .T. ) ;
#11330=ORIENTED_EDGE ( 'NONE', *, *, #2379, .T. ) ;
#11355=FACE_OUTER_BOUND ( 'NONE', #15903, .T. ) ;
#11406=CIRCLE ( 'NONE', #30012, 13.38408793869266411 ) ;
#11412=ORIENTED_EDGE ( 'NONE', *, *, #23100, .F. ) ;
#11451=ORIENTED_EDGE ( 'NONE', *, *, #22718, .F. ) ;
#11455=ORIENTED_EDGE ( 'NONE', *, *, #3289, .T. ) ;
#11565=AXIS2_PLACEMENT_3D ( 'NONE', #4244, #14718, #20384 ) ;
#11591=AXIS2_PLACEMENT_3D ( 'NONE', #19533, #32881, #17128 ) ;
#11609=CARTESIAN_POINT ( 'NONE',  ( 24.49999999999999645, -16.99999999999999289, 0.000000000000000000 ) ) ;
#11647=CARTESIAN_POINT ( 'NONE',  ( 4.349545668204547685E-15, -58.51673569255127205, 0.000000000000000000 ) ) ;
#11660=ORIENTED_EDGE ( 'NONE', *, *, #33984, .F. ) ;
#11667=EDGE_CURVE ( 'NONE', #19806, #30412, #5817, .T. ) ;
#11797=FACE_OUTER_BOUND ( 'NONE', #12636, .T. ) ;
#11826=ORIENTED_EDGE ( 'NONE', *, *, #27766, .F. ) ;
#11830=VERTEX_POINT ( 'NONE', #32312 ) ;
#11873=EDGE_CURVE ( 'NONE', #12231, #16950, #16880, .T. ) ;
#11882=CONICAL_SURFACE ( 'NONE', #26672, 15.31642273298461276, 0.2613323016132377830 ) ;
#11910=DIRECTION ( 'NONE',  ( -1.224646799147353454E-16, 1.000000000000000000, -0.000000000000000000 ) ) ;
#11978=DIRECTION ( 'NONE',  ( -1.224646799147353454E-16, 1.000000000000000000, -0.000000000000000000 ) ) ;
#12029=EDGE_CURVE ( 'NONE', #30412, #17976, #22525, .T. ) ;
#12050=DIRECTION ( 'NONE',  ( -1.224646799147353454E-16, 1.000000000000000000, -0.000000000000000000 ) ) ;
#12099=CARTESIAN_POINT ( 'NONE',  ( 26.49999999999999645, -1.999999999999995337, 3.245314017740485765E-15 ) ) ;
#12113=SURFACE_STYLE_FILL_AREA ( #20022 ) ;
#12123=CIRCLE ( 'NONE', #32933, 2.000000000000000000 ) ;
#12161=EDGE_CURVE ( 'NONE', #24826, #6369, #14981, .T. ) ;
#12165=LINE ( 'NONE', #33091, #16529 ) ;
#12216=CIRCLE ( 'NONE', #19362, 12.11000150615021909 ) ;
#12219=AXIS2_PLACEMENT_3D ( 'NONE', #21330, #24068, #31771 ) ;
#12231=VERTEX_POINT ( 'NONE', #28191 ) ;
#12247=DIRECTION ( 'NONE',  ( 1.000000000000000000, 0.000000000000000000, 0.000000000000000000 ) ) ;
#12281=DIRECTION ( 'NONE',  ( -1.000000000000000000, -1.416100796715761110E-16, 0.000000000000000000 ) ) ;
#12292=ADVANCED_FACE ( 'NONE', ( #5021 ), #20633, .F. ) ;
#12307=DIRECTION ( 'NONE',  ( 0.000000000000000000, -0.000000000000000000, -1.000000000000000000 ) ) ;
#12323=CARTESIAN_POINT ( 'NONE',  ( 8.327598234202002696E-15, -91.00000000000000000, 0.000000000000000000 ) ) ;
#12328=FACE_OUTER_BOUND ( 'NONE', #25409, .T. ) ;
#12342=DIRECTION ( 'NONE',  ( 1.000000000000000000, 0.000000000000000000, 0.000000000000000000 ) ) ;
#12408=EDGE_LOOP ( 'NONE', ( #20853, #14331 ) ) ;
#12431=ORIENTED_EDGE ( 'NONE', *, *, #18609, .F. ) ;
#12482=CARTESIAN_POINT ( 'NONE',  ( -2.571758278209442450E-15, -1.999999999999998224, 0.000000000000000000 ) ) ;
#12509=DIRECTION ( 'NONE',  ( -1.000000000000000000, 0.000000000000000000, 0.000000000000000000 ) ) ;
#12512=ADVANCED_FACE ( 'NONE', ( #30592 ), #8908, .T. ) ;
#12522=FACE_OUTER_BOUND ( 'NONE', #12408, .T. ) ;
#12538=EDGE_LOOP ( 'NONE', ( #31169, #32586, #11044, #24131 ) ) ;
#12579=EDGE_LOOP ( 'NONE', ( #18359, #266, #2690, #10117 ) ) ;
#12612=CARTESIAN_POINT ( 'NONE',  ( 3.469446951953614189E-15, -57.99999999999999289, 0.000000000000000000 ) ) ;
#12636=EDGE_LOOP ( 'NONE', ( #6701, #15535, #20726, #21888 ) ) ;
#12638=ORIENTED_EDGE ( 'NONE', *, *, #26046, .T. ) ;
#12678=CONICAL_SURFACE ( 'NONE', #23666, 15.31642273298461276, 0.2613323016132377830 ) ;
#12691=FACE_BOUND ( 'NONE', #28503, .T. ) ;
#12707=DIRECTION ( 'NONE',  ( -1.224646799147353454E-16, 1.000000000000000000, -0.000000000000000000 ) ) ;
#12714=DIRECTION ( 'NONE',  ( -1.224646799147353207E-16, -1.499759782661857882E-32, 1.000000000000000000 ) ) ;
#12752=AXIS2_PLACEMENT_3D ( 'NONE', #4539, #1608, #15012 ) ;
#12754=ORIENTED_EDGE ( 'NONE', *, *, #15316, .T. ) ;
#12840=DIRECTION ( 'NONE',  ( -1.000000000000000000, -1.224646799147353454E-16, 0.000000000000000000 ) ) ;
#12842=CARTESIAN_POINT ( 'NONE',  ( -15.31593959127081028, -56.96472381958990638, 0.000000000000000000 ) ) ;
#12862=DIRECTION ( 'NONE',  ( 1.000000000000000000, 1.224646799147353454E-16, 0.000000000000000000 ) ) ;
#12866=CARTESIAN_POINT ( 'NONE',  ( 4.412827539393359662E-15, -59.03347138510255832, 0.000000000000000000 ) ) ;
#12870=SURFACE_STYLE_USAGE ( .BOTH. , #2402 ) ;
#12898=ORIENTED_EDGE ( 'NONE', *, *, #3757, .F. ) ;
#12921=ORIENTED_EDGE ( 'NONE', *, *, #22774, .F. ) ;
#12937=EDGE_CURVE ( 'NONE', #19806, #28529, #4430, .T. ) ;
#12941=LINE ( 'NONE', #20847, #32148 ) ;
#12944=ORIENTED_EDGE ( 'NONE', *, *, #1897, .F. ) ;
#12946=EDGE_CURVE ( 'NONE', #7457, #23226, #30832, .T. ) ;
#12948=ORIENTED_EDGE ( 'NONE', *, *, #21821, .F. ) ;
#12978=CIRCLE ( 'NONE', #13548, 2.000000000000000000 ) ;
#12983=ORIENTED_EDGE ( 'NONE', *, *, #24210, .F. ) ;
#12986=ADVANCED_FACE ( 'NONE', ( #12328 ), #16595, .T. ) ;
#12988=ORIENTED_EDGE ( 'NONE', *, *, #15037, .T. ) ;
#13006=DIRECTION ( 'NONE',  ( -1.000000000000000000, 0.000000000000000000, 0.000000000000000000 ) ) ;
#13026=ORIENTED_EDGE ( 'NONE', *, *, #22774, .T. ) ;
#13072=EDGE_CURVE ( 'NONE', #20157, #4399, #4531, .T. ) ;
#13116=ORIENTED_EDGE ( 'NONE', *, *, #23213, .F. ) ;
#13145=ORIENTED_EDGE ( 'NONE', *, *, #17449, .F. ) ;
#13177=DIRECTION ( 'NONE',  ( -1.224646799147353454E-16, 1.000000000000000000, -0.000000000000000000 ) ) ;
#13204=( NAMED_UNIT ( * ) PLANE_ANGLE_UNIT ( ) SI_UNIT ( $, .RADIAN. ) );
#13215=EDGE_CURVE ( 'NONE', #9464, #1088, #136, .T. ) ;
#13217=CARTESIAN_POINT ( 'NONE',  ( 8.327598234202002696E-15, -91.00000000000000000, 0.000000000000000000 ) ) ;
#13245=VECTOR ( 'NONE', #5312, 1000.000000000000227 ) ;
#13313=VECTOR ( 'NONE', #1163, 1000.000000000000114 ) ;
#13315=DIRECTION ( 'NONE',  ( -1.000000000000000000, -1.224646799147353454E-16, 0.000000000000000000 ) ) ;
#13317=AXIS2_PLACEMENT_3D ( 'NONE', #7922, #5007, #15490 ) ;
#13326=DIRECTION ( 'NONE',  ( -1.224646799147353454E-16, 1.000000000000000000, -0.000000000000000000 ) ) ;
#13365=TOROIDAL_SURFACE ( 'NONE', #6756, 30.16025403784430736, 1.500000000000010436 ) ;
#13374=ORIENTED_EDGE ( 'NONE', *, *, #22144, .F. ) ;
#13387=AXIS2_PLACEMENT_3D ( 'NONE', #1766, #30776, #12247 ) ;
#13408=( GEOMETRIC_REPRESENTATION_CONTEXT ( 3 ) GLOBAL_UNCERTAINTY_ASSIGNED_CONTEXT ( ( #26770 ) ) GLOBAL_UNIT_ASSIGNED_CONTEXT ( ( #24512, #14220, #32058 ) ) REPRESENTATION_CONTEXT ( 'NONE', 'WORKASPACE' ) );
#13411=ORIENTED_EDGE ( 'NONE', *, *, #18187, .T. ) ;
#13421=DIRECTION ( 'NONE',  ( -1.000000000000000000, 0.000000000000000000, 0.000000000000000000 ) ) ;
#13437=VECTOR ( 'NONE', #3768, 1000.000000000000227 ) ;
#13454=TOROIDAL_SURFACE ( 'NONE', #32601, 30.16025403784430736, 3.500000000000010658 ) ;
#13548=AXIS2_PLACEMENT_3D ( 'NONE', #24237, #708, #32110 ) ;
#13557=CIRCLE ( 'NONE', #3143, 4.000000000000014211 ) ;
#13581=CIRCLE ( 'NONE', #2601, 26.50000000000000000 ) ;
#13609=AXIS2_PLACEMENT_3D ( 'NONE', #31973, #13637, #24101 ) ;
#13637=DIRECTION ( 'NONE',  ( 0.000000000000000000, -0.000000000000000000, -1.000000000000000000 ) ) ;
#13680=DIRECTION ( 'NONE',  ( -1.000000000000000000, 0.000000000000000000, 0.000000000000000000 ) ) ;
#13703=VERTEX_POINT ( 'NONE', #6336 ) ;
#13746=FACE_OUTER_BOUND ( 'NONE', #23918, .T. ) ;
#13749=PRODUCT_DEFINITION_SHAPE ( 'NONE', 'NONE',  #8255 ) ;
#13767=CARTESIAN_POINT ( 'NONE',  ( 10.72870458603808785, -72.44024934668307480, 1.313887373028906799E-15 ) ) ;
#13833=ORIENTED_EDGE ( 'NONE', *, *, #32348, .F. ) ;
#13902=LINE ( 'NONE', #24693, #25822 ) ;
#13920=DIRECTION ( 'NONE',  ( 1.000000000000000000, 0.000000000000000000, 0.000000000000000000 ) ) ;
#13967=CARTESIAN_POINT ( 'NONE',  ( 7.428728520588063561E-18, -23.06066017177981564, 0.000000000000000000 ) ) ;
#13989=ADVANCED_FACE ( 'NONE', ( #1165 ), #9441, .F. ) ;
#14067=DIRECTION ( 'NONE',  ( -1.000000000000000000, 0.000000000000000000, 0.000000000000000000 ) ) ;
#14117=ADVANCED_FACE ( 'NONE', ( #27603 ), #16619, .T. ) ;
#14220=( NAMED_UNIT ( * ) PLANE_ANGLE_UNIT ( ) SI_UNIT ( $, .RADIAN. ) );
#14239=LINE ( 'NONE', #27275, #13437 ) ;
#14291=CARTESIAN_POINT ( 'NONE',  ( -2.571758278209442450E-15, -1.999999999999998224, 0.000000000000000000 ) ) ;
#14309=VECTOR ( 'NONE', #8156, 1000.000000000000227 ) ;
#14331=ORIENTED_EDGE ( 'NONE', *, *, #9080, .T. ) ;
#14342=CIRCLE ( 'NONE', #32957, 10.69578794377714104 ) ;
#14385=CONICAL_SURFACE ( 'NONE', #3970, 24.50000000000000000, 0.7853981633974463916 ) ;
#14394=ADVANCED_FACE ( 'NONE', ( #20757 ), #28661, .T. ) ;
#14499=ORIENTED_EDGE ( 'NONE', *, *, #3289, .F. ) ;
#14512=CARTESIAN_POINT ( 'NONE',  ( 4.349545668204547685E-15, -58.51673569255127205, 0.000000000000000000 ) ) ;
#14529=( NAMED_UNIT ( * ) SI_UNIT ( $, .STERADIAN. ) SOLID_ANGLE_UNIT ( ) );
#14660=ORIENTED_EDGE ( 'NONE', *, *, #29841, .F. ) ;
#14718=DIRECTION ( 'NONE',  ( -1.224646799147353454E-16, 1.000000000000000000, -0.000000000000000000 ) ) ;
#14793=ORIENTED_EDGE ( 'NONE', *, *, #28085, .F. ) ;
#14809=PRODUCT_DEFINITION_FORMATION_WITH_SPECIFIED_SOURCE ( 'ANY', '', #4952, .NOT_KNOWN. ) ;
#14830=EDGE_CURVE ( 'NONE', #27878, #19445, #12216, .T. ) ;
#14831=FACE_OUTER_BOUND ( 'NONE', #2481, .T. ) ;
#14839=DIRECTION ( 'NONE',  ( -1.224646799147353454E-16, 1.000000000000000000, -0.000000000000000000 ) ) ;
#14880=CIRCLE ( 'NONE', #29656, 10.17814985357208890 ) ;
#14881=TOROIDAL_SURFACE ( 'NONE', #27467, 11.45223628611452860, 4.000000000000014211 ) ;
#14916=VERTEX_POINT ( 'NONE', #21634 ) ;
#14953=AXIS2_PLACEMENT_3D ( 'NONE', #14291, #19446, #9643 ) ;
#14959=CARTESIAN_POINT ( 'NONE',  ( 30.91025403784432868, -20.70096189432334199, 0.000000000000000000 ) ) ;
#14981=LINE ( 'NONE', #4507, #10212 ) ;
#15012=DIRECTION ( 'NONE',  ( -1.000000000000000000, 0.000000000000000000, 0.000000000000000000 ) ) ;
#15022=CONICAL_SURFACE ( 'NONE', #13387, 10.17814985357208890, 0.2617993877991527385 ) ;
#15037=EDGE_CURVE ( 'NONE', #14916, #5385, #19889, .T. ) ;
#15086=DIRECTION ( 'NONE',  ( -1.000000000000000000, -1.145572106777136737E-16, 0.000000000000000000 ) ) ;
#15122=ADVANCED_FACE ( 'NONE', ( #281 ), #7838, .T. ) ;
#15178=ORIENTED_EDGE ( 'NONE', *, *, #15316, .F. ) ;
#15184=VERTEX_POINT ( 'NONE', #31354 ) ;
#15187=ORIENTED_EDGE ( 'NONE', *, *, #32622, .F. ) ;
#15223=DIRECTION ( 'NONE',  ( -1.000000000000000000, -1.063101997391471025E-16, 0.000000000000000000 ) ) ;
#15260=ADVANCED_BREP_SHAPE_REPRESENTATION ( '', ( #33133, #1376 ), #231 ) ;
#15316=EDGE_CURVE ( 'NONE', #18620, #15868, #374, .T. ) ;
#15332=DIRECTION ( 'NONE',  ( -1.224646799147353454E-16, 1.000000000000000000, -0.000000000000000000 ) ) ;
#15362=ORIENTED_EDGE ( 'NONE', *, *, #27766, .T. ) ;
#15425=DIRECTION ( 'NONE',  ( -1.224646799147353454E-16, 1.000000000000000000, -0.000000000000000000 ) ) ;
#15439=ORIENTED_EDGE ( 'NONE', *, *, #27464, .T. ) ;
#15490=DIRECTION ( 'NONE',  ( 1.000000000000000000, 0.000000000000000000, 1.224646799147352714E-16 ) ) ;
#15535=ORIENTED_EDGE ( 'NONE', *, *, #24657, .T. ) ;
#15573=ORIENTED_EDGE ( 'NONE', *, *, #29737, .T. ) ;
#15575=CARTESIAN_POINT ( 'NONE',  ( 1.806199397676865774E-16, -24.47487373415291145, 0.000000000000000000 ) ) ;
#15584=DIRECTION ( 'NONE',  ( -1.000000000000000000, 0.000000000000000000, 0.000000000000000000 ) ) ;
#15686=CONICAL_SURFACE ( 'NONE', #3608, 26.50000000000000000, 1.047197551196594523 ) ;
#15697=ORIENTED_EDGE ( 'NONE', *, *, #7258, .F. ) ;
#15760=DIRECTION ( 'NONE',  ( -1.000000000000000000, 0.000000000000000000, 0.000000000000000000 ) ) ;
#15763=DIRECTION ( 'NONE',  ( -1.224646799147353454E-16, 1.000000000000000000, -0.000000000000000000 ) ) ;
#15792=ADVANCED_FACE ( 'NONE', ( #24971 ), #26695, .F. ) ;
#15825=EDGE_LOOP ( 'NONE', ( #23582, #25260, #27641, #12983 ) ) ;
#15829=DIRECTION ( 'NONE',  ( -1.224646799147353454E-16, 1.000000000000000000, -0.000000000000000000 ) ) ;
#15835=LINE ( 'NONE', #20818, #22754 ) ;
#15865=LINE ( 'NONE', #21352, #6409 ) ;
#15868=VERTEX_POINT ( 'NONE', #13767 ) ;
#15903=EDGE_LOOP ( 'NONE', ( #15573, #25298, #22938, #11293 ) ) ;
#15927=DIRECTION ( 'NONE',  ( -1.224646799147353454E-16, 1.000000000000000000, -0.000000000000000000 ) ) ;
#16072=AXIS2_PLACEMENT_3D ( 'NONE', #4708, #20514, #7279 ) ;
#16089=EDGE_CURVE ( 'NONE', #20029, #25648, #27762, .T. ) ;
#16100=CARTESIAN_POINT ( 'NONE',  ( 3.469446951953614189E-15, -45.00000000000000000, 0.000000000000000000 ) ) ;
#16101=CARTESIAN_POINT ( 'NONE',  ( -24.50000000000000000, -29.78157438140398838, 0.000000000000000000 ) ) ;
#16109=LINE ( 'NONE', #21255, #31951 ) ;
#16111=CARTESIAN_POINT ( 'NONE',  ( -11.45223628611452504, -57.99999999999999289, 0.000000000000000000 ) ) ;
#16128=CARTESIAN_POINT ( 'NONE',  ( 3.469446951953614189E-15, -45.00000000000000000, 0.000000000000000000 ) ) ;
#16152=DIRECTION ( 'NONE',  ( -1.000000000000000000, 0.000000000000000000, 0.000000000000000000 ) ) ;
#16156=DIRECTION ( 'NONE',  ( -1.000000000000000000, 0.000000000000000000, 0.000000000000000000 ) ) ;
#16178=EDGE_CURVE ( 'NONE', #6976, #18620, #12978, .T. ) ;
#16184=ADVANCED_FACE ( 'NONE', ( #11355 ), #11882, .T. ) ;
#16201=CARTESIAN_POINT ( 'NONE',  ( 0.000000000000000000, -23.00000000000000000, 0.000000000000000000 ) ) ;
#16202=ORIENTED_EDGE ( 'NONE', *, *, #32222, .F. ) ;
#16223=AXIS2_PLACEMENT_3D ( 'NONE', #25504, #4221, #12281 ) ;
#16243=VECTOR ( 'NONE', #4169, 1000.000000000000227 ) ;
#16248=DIRECTION ( 'NONE',  ( -0.7202789989107549751, -0.6936844842780617304, 8.820873705091161919E-17 ) ) ;
#16274=AXIS2_PLACEMENT_3D ( 'NONE', #3963, #11194, #24892 ) ;
#16309=DIRECTION ( 'NONE',  ( -1.224646799147353454E-16, 1.000000000000000000, -0.000000000000000000 ) ) ;
#16316=CARTESIAN_POINT ( 'NONE',  ( -12.11607355459419821, -70.99969134886156041, 1.483791069686768580E-15 ) ) ;
#16320=DIRECTION ( 'NONE',  ( -1.224646799147353454E-16, 1.000000000000000000, -0.000000000000000000 ) ) ;
#16484=CARTESIAN_POINT ( 'NONE',  ( 11.45223628611453215, -57.99999999999999289, 1.402494451086933009E-15 ) ) ;
#16520=AXIS2_PLACEMENT_3D ( 'NONE', #21816, #3450, #13920 ) ;
#16528=CIRCLE ( 'NONE', #7752, 2.000000000000000000 ) ;
#16529=VECTOR ( 'NONE', #9594, 1000.000000000000114 ) ;
#16595=CONICAL_SURFACE ( 'NONE', #25894, 32.63512777199724724, 0.7853981633974471688 ) ;
#16619=TOROIDAL_SURFACE ( 'NONE', #6190, 12.11000150615021553, 1.999999999999992228 ) ;
#16626=FACE_OUTER_BOUND ( 'NONE', #7533, .T. ) ;
#16842=DIRECTION ( 'NONE',  ( -1.000000000000000000, -1.122425893913996568E-16, 0.000000000000000000 ) ) ;
#16861=CARTESIAN_POINT ( 'NONE',  ( 5.878266837044421923E-15, -70.99969134886156041, 0.000000000000000000 ) ) ;
#16868=ORIENTED_EDGE ( 'NONE', *, *, #23060, .F. ) ;
#16880=LINE ( 'NONE', #16101, #6905 ) ;
#16950=VERTEX_POINT ( 'NONE', #7857 ) ;
#17021=ADVANCED_FACE ( 'NONE', ( #7689 ), #2013, .T. ) ;
#17048=CARTESIAN_POINT ( 'NONE',  ( 30.16025403784430736, -21.99999999999999289, 3.693565856891707127E-15 ) ) ;
#17065=AXIS2_PLACEMENT_3D ( 'NONE', #5430, #13326, #23799 ) ;
#17122=EDGE_CURVE ( 'NONE', #6224, #29257, #6398, .T. ) ;
#17128=DIRECTION ( 'NONE',  ( -1.000000000000000000, -1.309225264888156377E-16, 0.000000000000000000 ) ) ;
#17136=TOROIDAL_SURFACE ( 'NONE', #19340, 11.45223628611452860, 2.000000000000014211 ) ;
#17149=DIRECTION ( 'NONE',  ( -1.000000000000000000, 0.000000000000000000, 0.000000000000000000 ) ) ;
#17183=AXIS2_PLACEMENT_3D ( 'NONE', #2593, #12714, #10316 ) ;
#17238=ORIENTED_EDGE ( 'NONE', *, *, #7688, .F. ) ;
#17250=FACE_OUTER_BOUND ( 'NONE', #12579, .T. ) ;
#17276=SURFACE_SIDE_STYLE ('',( #12113 ) ) ;
#17313=CARTESIAN_POINT ( 'NONE',  ( 10.17814985357209245, -45.51763809020504681, 0.000000000000000000 ) ) ;
#17330=CIRCLE ( 'NONE', #6780, 26.50000000000000000 ) ;
#17358=AXIS2_PLACEMENT_3D ( 'NONE', #14512, #9344, #19827 ) ;
#17364=AXIS2_PLACEMENT_3D ( 'NONE', #6593, #11910, #27529 ) ;
#17408=ADVANCED_FACE ( 'NONE', ( #24982 ), #32696, .F. ) ;
#17449=EDGE_CURVE ( 'NONE', #21971, #31380, #19675, .T. ) ;
#17586=ORIENTED_EDGE ( 'NONE', *, *, #6380, .T. ) ;
#17589=DIRECTION ( 'NONE',  ( -1.000000000000000000, -1.416100796715760863E-16, 0.000000000000000000 ) ) ;
#17629=CARTESIAN_POINT ( 'NONE',  ( 12.11000150615021909, -45.00000000000000000, 1.483047458217648827E-15 ) ) ;
#17654=CARTESIAN_POINT ( 'NONE',  ( 4.159479030958464888E-15, -56.96472381958990638, 0.000000000000000000 ) ) ;
#17669=ORIENTED_EDGE ( 'NONE', *, *, #33593, .F. ) ;
#17689=CARTESIAN_POINT ( 'NONE',  ( -8.761981113183991350E-16, -15.84529946162075298, 0.000000000000000000 ) ) ;
#17725=AXIS2_PLACEMENT_3D ( 'NONE', #15575, #18149, #15223 ) ;
#17729=CARTESIAN_POINT ( 'NONE',  ( 12.11607355459420710, -70.99969134886156041, 1.483791069686768383E-15 ) ) ;
#17774=DIRECTION ( 'NONE',  ( -1.000000000000000000, -1.309225264888156377E-16, 0.000000000000000000 ) ) ;
#17841=EDGE_CURVE ( 'NONE', #23226, #4399, #253, .T. ) ;
#17884=CONICAL_SURFACE ( 'NONE', #32620, 26.50000000000000000, 1.047197551196594523 ) ;
#17906=CARTESIAN_POINT ( 'NONE',  ( 12.11607355459420710, -70.99969134886156041, 1.483791069686768383E-15 ) ) ;
#17941=EDGE_LOOP ( 'NONE', ( #27028, #14660, #10712, #24294 ) ) ;
#17976=VERTEX_POINT ( 'NONE', #27186 ) ;
#17988=DIRECTION ( 'NONE',  ( -1.000000000000000000, -1.145572106777136737E-16, 0.000000000000000000 ) ) ;
#18004=DIRECTION ( 'NONE',  ( -1.000000000000000000, -1.063101997391471025E-16, 0.000000000000000000 ) ) ;
#18020=ORIENTED_EDGE ( 'NONE', *, *, #13072, .F. ) ;
#18102=ORIENTED_EDGE ( 'NONE', *, *, #28135, .T. ) ;
#18149=DIRECTION ( 'NONE',  ( -1.224646799147353454E-16, 1.000000000000000000, -0.000000000000000000 ) ) ;
#18174=CARTESIAN_POINT ( 'NONE',  ( 5.204170427930421283E-15, -70.99969134886156041, 0.000000000000000000 ) ) ;
#18185=AXIS2_PLACEMENT_3D ( 'NONE', #28953, #10093, #13006 ) ;
#18187=EDGE_CURVE ( 'NONE', #13703, #7411, #23786, .T. ) ;
#18204=FILL_AREA_STYLE_COLOUR ( '', #24355 ) ;
#18232=ORIENTED_EDGE ( 'NONE', *, *, #30542, .F. ) ;
#18239=DIRECTION ( 'NONE',  ( -1.224646799147353454E-16, 1.000000000000000000, -0.000000000000000000 ) ) ;
#18256=ORIENTED_EDGE ( 'NONE', *, *, #27274, .T. ) ;
#18270=ORIENTED_EDGE ( 'NONE', *, *, #23296, .F. ) ;
#18312=EDGE_CURVE ( 'NONE', #19445, #11212, #33473, .T. ) ;
#18330=CARTESIAN_POINT ( 'NONE',  ( -32.63512777199724724, -24.47487373415291501, 0.000000000000000000 ) ) ;
#18359=ORIENTED_EDGE ( 'NONE', *, *, #27039, .F. ) ;
#18370=FACE_OUTER_BOUND ( 'NONE', #18698, .T. ) ;
#18450=ORIENTED_EDGE ( 'NONE', *, *, #30542, .T. ) ;
#18528=ORIENTED_EDGE ( 'NONE', *, *, #27464, .F. ) ;
#18532=ORIENTED_EDGE ( 'NONE', *, *, #6380, .F. ) ;
#18571=ORIENTED_EDGE ( 'NONE', *, *, #6845, .T. ) ;
#18609=EDGE_CURVE ( 'NONE', #23226, #11830, #13902, .T. ) ;
#18613=CARTESIAN_POINT ( 'NONE',  ( -13.38432950954956624, -58.51673569255127205, 0.000000000000000000 ) ) ;
#18616=ORIENTED_EDGE ( 'NONE', *, *, #7565, .F. ) ;
#18620=VERTEX_POINT ( 'NONE', #22297 ) ;
#18668=CARTESIAN_POINT ( 'NONE',  ( 2.694222958124179176E-15, -45.00000000000001421, 0.000000000000000000 ) ) ;
#18698=EDGE_LOOP ( 'NONE', ( #26783, #1054, #4665, #18232 ) ) ;
#18755=FACE_OUTER_BOUND ( 'NONE', #11083, .T. ) ;
#18784=CARTESIAN_POINT ( 'NONE',  ( -12.11000150615021198, -45.00000000000000000, 0.000000000000000000 ) ) ;
#18810=DIRECTION ( 'NONE',  ( -1.224646799147353454E-16, 1.000000000000000000, -0.000000000000000000 ) ) ;
#18856=CIRCLE ( 'NONE', #6220, 13.38408793869266411 ) ;
#18868=DIRECTION ( 'NONE',  ( 1.000000000000000000, 0.000000000000000000, 0.000000000000000000 ) ) ;
#18896=ORIENTED_EDGE ( 'NONE', *, *, #23201, .T. ) ;
#18905=CARTESIAN_POINT ( 'NONE',  ( 8.305033359366087120E-16, -29.78157438140398483, 0.000000000000000000 ) ) ;
#18926=AXIS2_PLACEMENT_3D ( 'NONE', #22457, #2034, #12509 ) ;
#18981=ORIENTED_EDGE ( 'NONE', *, *, #18609, .T. ) ;
#18990=EDGE_LOOP ( 'NONE', ( #25306, #31290, #4915, #14499 ) ) ;
#19000=DIRECTION ( 'NONE',  ( -1.224646799147353454E-16, 1.000000000000000000, -0.000000000000000000 ) ) ;
#19015=AXIS2_PLACEMENT_3D ( 'NONE', #7677, #31524, #15760 ) ;
#19056=DIRECTION ( 'NONE',  ( -1.224646799147353454E-16, 1.000000000000000000, -0.000000000000000000 ) ) ;
#19092=CARTESIAN_POINT ( 'NONE',  ( 4.412827539393359662E-15, -59.03347138510255832, 0.000000000000000000 ) ) ;
#19189=ORIENTED_EDGE ( 'NONE', *, *, #28085, .T. ) ;
#19232=ORIENTED_EDGE ( 'NONE', *, *, #10938, .F. ) ;
#19273=ORIENTED_EDGE ( 'NONE', *, *, #28135, .F. ) ;
#19306=FACE_OUTER_BOUND ( 'NONE', #23071, .T. ) ;
#19318=ORIENTED_EDGE ( 'NONE', *, *, #12937, .T. ) ;
#19335=AXIS2_PLACEMENT_3D ( 'NONE', #17654, #15425, #4602 ) ;
#19340=AXIS2_PLACEMENT_3D ( 'NONE', #31258, #28351, #7751 ) ;
#19362=AXIS2_PLACEMENT_3D ( 'NONE', #21799, #16320, #16156 ) ;
#19445=VERTEX_POINT ( 'NONE', #24163 ) ;
#19446=DIRECTION ( 'NONE',  ( -1.224646799147353454E-16, 1.000000000000000000, -0.000000000000000000 ) ) ;
#19533=CARTESIAN_POINT ( 'NONE',  ( 0.000000000000000000, -23.00000000000000000, 0.000000000000000000 ) ) ;
#19552=PRODUCT_DEFINITION_CONTEXT ( 'detailed design', #4386, 'design' ) ;
#19565=DIRECTION ( 'NONE',  ( -1.224646799147353454E-16, 1.000000000000000000, -0.000000000000000000 ) ) ;
#19566=EDGE_LOOP ( 'NONE', ( #32632, #1032, #1996, #10291 ) ) ;
#19642=EDGE_CURVE ( 'NONE', #7457, #20157, #3554, .T. ) ;
#19675=LINE ( 'NONE', #22411, #4144 ) ;
#19696=SHAPE_REPRESENTATION ( 'bellows suction cup', ( #1376 ), #231 ) ;
#19715=CARTESIAN_POINT ( 'NONE',  ( -7.347880794884122694E-16, -16.99999999999999645, 0.000000000000000000 ) ) ;
#19774=CIRCLE ( 'NONE', #24173, 32.63512777199724724 ) ;
#19806=VERTEX_POINT ( 'NONE', #30466 ) ;
#19811=ORIENTED_EDGE ( 'NONE', *, *, #5178, .F. ) ;
#19827=DIRECTION ( 'NONE',  ( -1.000000000000000000, 0.000000000000000000, 0.000000000000000000 ) ) ;
#19835=DIRECTION ( 'NONE',  ( -1.000000000000000000, -1.224646799147353454E-16, 0.000000000000000000 ) ) ;
#19883=DIRECTION ( 'NONE',  ( -1.000000000000000000, -1.224646799147353454E-16, 0.000000000000000000 ) ) ;
#19889=CIRCLE ( 'NONE', #3455, 31.91025403784435710 ) ;
#19935=CARTESIAN_POINT ( 'NONE',  ( -15.31642273298460744, -59.03347138510255832, 0.000000000000000000 ) ) ;
#20013=DIRECTION ( 'NONE',  ( -1.224646799147353454E-16, 1.000000000000000000, -0.000000000000000000 ) ) ;
#20022=FILL_AREA_STYLE ('',( #3890 ) ) ;
#20029=VERTEX_POINT ( 'NONE', #19935 ) ;
#20056=CARTESIAN_POINT ( 'NONE',  ( -12.11607355459419821, -70.99969134886156041, 2.663817581893346643E-15 ) ) ;
#20093=DIRECTION ( 'NONE',  ( -0.7071067811865467956, 0.7071067811865483499, 0.000000000000000000 ) ) ;
#20157=VERTEX_POINT ( 'NONE', #14959 ) ;
#20200=EDGE_LOOP ( 'NONE', ( #16868, #13411, #26195, #28972 ) ) ;
#20265=CARTESIAN_POINT ( 'NONE',  ( 5.204170427930421283E-15, -70.99969134886156041, 0.000000000000000000 ) ) ;
#20294=DIRECTION ( 'NONE',  ( -1.000000000000000000, -1.416100796715761110E-16, 0.000000000000000000 ) ) ;
#20332=ORIENTED_EDGE ( 'NONE', *, *, #30392, .T. ) ;
#20342=DIRECTION ( 'NONE',  ( -1.224646799147353454E-16, 1.000000000000000000, -0.000000000000000000 ) ) ;
#20354=AXIS2_PLACEMENT_3D ( 'NONE', #26546, #27674, #29604 ) ;
#20355=CONICAL_SURFACE ( 'NONE', #24201, 12.11000150615021909, 0.2617993877991545149 ) ;
#20384=DIRECTION ( 'NONE',  ( -1.000000000000000000, 0.000000000000000000, 0.000000000000000000 ) ) ;
#20472=CIRCLE ( 'NONE', #5672, 10.18398033115917656 ) ;
#20514=DIRECTION ( 'NONE',  ( -1.224646799147353454E-16, 1.000000000000000000, -0.000000000000000000 ) ) ;
#20553=FACE_OUTER_BOUND ( 'NONE', #12538, .T. ) ;
#20555=DIRECTION ( 'NONE',  ( -1.224646799147353207E-16, -1.499759782661857882E-32, 1.000000000000000000 ) ) ;
#20577=DIRECTION ( 'NONE',  ( -1.000000000000000000, 0.000000000000000000, 0.000000000000000000 ) ) ;
#20580=CARTESIAN_POINT ( 'NONE',  ( 8.327598234202002696E-15, -91.00000000000000000, 0.000000000000000000 ) ) ;
#20595=FACE_OUTER_BOUND ( 'NONE', #23206, .T. ) ;
#20608=LINE ( 'NONE', #28815, #13245 ) ;
#20617=FACE_OUTER_BOUND ( 'NONE', #10625, .T. ) ;
#20633=TOROIDAL_SURFACE ( 'NONE', #29375, 30.16025403784430736, 1.500000000000010436 ) ;
#20637=DIRECTION ( 'NONE',  ( -1.000000000000000000, 0.000000000000000000, 0.000000000000000000 ) ) ;
#20666=ORIENTED_EDGE ( 'NONE', *, *, #19642, .T. ) ;
#20671=EDGE_CURVE ( 'NONE', #21883, #5385, #23656, .T. ) ;
#20689=ORIENTED_EDGE ( 'NONE', *, *, #12937, .F. ) ;
#20726=ORIENTED_EDGE ( 'NONE', *, *, #4609, .T. ) ;
#20739=CARTESIAN_POINT ( 'NONE',  ( 12.11607355459420887, -70.99969134886156041, 0.000000000000000000 ) ) ;
#20757=FACE_OUTER_BOUND ( 'NONE', #11291, .T. ) ;
#20758=DIRECTION ( 'NONE',  ( -1.000000000000000000, -1.224646799147353454E-16, 0.000000000000000000 ) ) ;
#20818=CARTESIAN_POINT ( 'NONE',  ( -26.50000000000000000, -15.84529946162075653, 3.245314017740485765E-15 ) ) ;
#20847=CARTESIAN_POINT ( 'NONE',  ( 30.00000000000001421, -91.00000000000000000, 3.673940397442059967E-15 ) ) ;
#20853=ORIENTED_EDGE ( 'NONE', *, *, #32622, .T. ) ;
#20889=ORIENTED_EDGE ( 'NONE', *, *, #22244, .T. ) ;
#20900=CIRCLE ( 'NONE', #11565, 10.72870458603808075 ) ;
#20916=DIRECTION ( 'NONE',  ( -1.224646799147353454E-16, 1.000000000000000000, -0.000000000000000000 ) ) ;
#20926=AXIS2_PLACEMENT_3D ( 'NONE', #8021, #15763, #7849 ) ;
#20927=CIRCLE ( 'NONE', #28037, 30.00000000000000711 ) ;
#20998=DIRECTION ( 'NONE',  ( -1.000000000000000000, 0.000000000000000000, 0.000000000000000000 ) ) ;
#21011=CARTESIAN_POINT ( 'NONE',  ( -7.347880794884122694E-16, -16.99999999999999645, 0.000000000000000000 ) ) ;
#21021=ADVANCED_FACE ( 'NONE', ( #26950 ), #30182, .T. ) ;
#21122=DIRECTION ( 'NONE',  ( -1.000000000000000000, -1.224646799147353454E-16, 0.000000000000000000 ) ) ;
#21126=DIRECTION ( 'NONE',  ( -1.224646799147353454E-16, 1.000000000000000000, -0.000000000000000000 ) ) ;
#21182=DIRECTION ( 'NONE',  ( -1.224646799147353454E-16, 1.000000000000000000, -0.000000000000000000 ) ) ;
#21222=AXIS2_PLACEMENT_3D ( 'NONE', #18174, #8195, #28617 ) ;
#21228=CIRCLE ( 'NONE', #7519, 10.11000150615022264 ) ;
#21255=CARTESIAN_POINT ( 'NONE',  ( -30.00000000000000000, -91.00000000000000000, 0.000000000000000000 ) ) ;
#21280=CIRCLE ( 'NONE', #13609, 1.500000000000008216 ) ;
#21330=CARTESIAN_POINT ( 'NONE',  ( 6.054684311146244891E-15, -72.44024934668307480, 0.000000000000000000 ) ) ;
#21352=CARTESIAN_POINT ( 'NONE',  ( 26.50000000000000000, -15.84529946162074943, 0.000000000000000000 ) ) ;
#21386=ORIENTED_EDGE ( 'NONE', *, *, #15037, .F. ) ;
#21444=DIRECTION ( 'NONE',  ( -1.000000000000000000, -1.224646799147353454E-16, 0.000000000000000000 ) ) ;
#21510=EDGE_LOOP ( 'NONE', ( #27813, #23503, #11170, #9483 ) ) ;
#21554=EDGE_LOOP ( 'NONE', ( #5645, #6007, #19318, #32135 ) ) ;
#21559=ORIENTED_EDGE ( 'NONE', *, *, #23100, .T. ) ;
#21619=TOROIDAL_SURFACE ( 'NONE', #237, 12.11000150615021553, 1.999999999999992228 ) ;
#21634=CARTESIAN_POINT ( 'NONE',  ( 31.91025403784435710, -18.96891108675447413, 3.952264761658314980E-15 ) ) ;
#21694=CARTESIAN_POINT ( 'NONE',  ( 30.16025403784430736, -21.99999999999999289, 3.693565856891707127E-15 ) ) ;
#21716=CARTESIAN_POINT ( 'NONE',  ( -24.49999999999999645, -17.00000000000000000, 3.000384657911015074E-15 ) ) ;
#21725=LINE ( 'NONE', #32171, #8131 ) ;
#21799=CARTESIAN_POINT ( 'NONE',  ( 2.694222958124179176E-15, -45.00000000000001421, 0.000000000000000000 ) ) ;
#21816=CARTESIAN_POINT ( 'NONE',  ( 5.878266837044421923E-15, -70.99969134886156041, 0.000000000000000000 ) ) ;
#21818=DIRECTION ( 'NONE',  ( 1.000000000000000000, 0.000000000000000000, 0.000000000000000000 ) ) ;
#21821=EDGE_CURVE ( 'NONE', #15868, #18620, #20900, .T. ) ;
#21883=VERTEX_POINT ( 'NONE', #18330 ) ;
#21888=ORIENTED_EDGE ( 'NONE', *, *, #9080, .F. ) ;
#21971=VERTEX_POINT ( 'NONE', #20739 ) ;
#21987=DIRECTION ( 'NONE',  ( 1.000000000000000000, 1.309225264888156377E-16, 0.000000000000000000 ) ) ;
#22128=CARTESIAN_POINT ( 'NONE',  ( 1.806199397676865774E-16, -24.47487373415291145, 0.000000000000000000 ) ) ;
#22144=EDGE_CURVE ( 'NONE', #19445, #27878, #28008, .T. ) ;
#22152=TOROIDAL_SURFACE ( 'NONE', #28174, 11.45223628611452860, 2.000000000000014211 ) ;
#22228=TOROIDAL_SURFACE ( 'NONE', #31553, 12.11607355459420177, 2.000000000000000000 ) ;
#22244=EDGE_CURVE ( 'NONE', #5385, #14916, #25337, .T. ) ;
#22259=SURFACE_STYLE_USAGE ( .BOTH. , #17276 ) ;
#22297=CARTESIAN_POINT ( 'NONE',  ( -10.72870458603807720, -72.44024934668307480, 0.000000000000000000 ) ) ;
#22324=CARTESIAN_POINT ( 'NONE',  ( -11.45223628611452504, -57.99999999999999289, 0.000000000000000000 ) ) ;
#22380=ORIENTED_EDGE ( 'NONE', *, *, #5286, .T. ) ;
#22411=CARTESIAN_POINT ( 'NONE',  ( 12.11607355459420887, -70.99969134886156041, 0.000000000000000000 ) ) ;
#22457=CARTESIAN_POINT ( 'NONE',  ( 8.151180760100182884E-15, -89.55944200217849982, 0.000000000000000000 ) ) ;
#22463=EDGE_CURVE ( 'NONE', #11212, #21883, #19774, .T. ) ;
#22483=DIRECTION ( 'NONE',  ( 1.224646799147353454E-16, -1.000000000000000000, 0.000000000000000000 ) ) ;
#22511=CARTESIAN_POINT ( 'NONE',  ( -12.11607355459419644, -70.99969134886156041, 0.000000000000000000 ) ) ;
#22525=LINE ( 'NONE', #6909, #16243 ) ;
#22585=( NAMED_UNIT ( * ) PLANE_ANGLE_UNIT ( ) SI_UNIT ( $, .RADIAN. ) );
#22685=AXIS2_PLACEMENT_3D ( 'NONE', #6574, #27000, #32147 ) ;
#22705=ORIENTED_EDGE ( 'NONE', *, *, #11667, .T. ) ;
#22708=MECHANICAL_DESIGN_GEOMETRIC_PRESENTATION_REPRESENTATION('',(#9540),#13408);
#22718=EDGE_CURVE ( 'NONE', #13703, #3977, #12123, .T. ) ;
#22754=VECTOR ( 'NONE', #5187, 1000.000000000000227 ) ;
#22761=PRESENTATION_STYLE_ASSIGNMENT (( #22259 ) ) ;
#22774=EDGE_CURVE ( 'NONE', #3977, #15868, #16528, .T. ) ;
#22795=CARTESIAN_POINT ( 'NONE',  ( -2.571758278209442450E-15, -1.999999999999998224, 0.000000000000000000 ) ) ;
#22798=DIRECTION ( 'NONE',  ( -1.000000000000000000, -1.063101997391471025E-16, 0.000000000000000000 ) ) ;
#22808=ORIENTED_EDGE ( 'NONE', *, *, #24210, .T. ) ;
#22811=FACE_OUTER_BOUND ( 'NONE', #1561, .T. ) ;
#22828=DIRECTION ( 'NONE',  ( 1.000000000000000000, 1.309225264888156377E-16, 0.000000000000000000 ) ) ;
#22849=CONICAL_SURFACE ( 'NONE', #27231, 12.11607355459420354, 0.8042044335707554392 ) ;
#22869=DIRECTION ( 'NONE',  ( -1.224646799147353207E-16, -1.499759782661857882E-32, 1.000000000000000000 ) ) ;
#22876=AXIS2_PLACEMENT_3D ( 'NONE', #18905, #15829, #29352 ) ;
#22938=ORIENTED_EDGE ( 'NONE', *, *, #16089, .F. ) ;
#22944=CARTESIAN_POINT ( 'NONE',  ( 5.878266837044421923E-15, -70.99969134886156041, 0.000000000000000000 ) ) ;
#23034=ORIENTED_EDGE ( 'NONE', *, *, #16178, .F. ) ;
#23060=EDGE_CURVE ( 'NONE', #13703, #24826, #1707, .T. ) ;
#23071=EDGE_LOOP ( 'NONE', ( #18528, #18571, #18102, #13116 ) ) ;
#23100=EDGE_CURVE ( 'NONE', #3977, #6976, #24199, .T. ) ;
#23106=VERTEX_POINT ( 'NONE', #23478 ) ;
#23110=CARTESIAN_POINT ( 'NONE',  ( 5.814984965855610735E-15, -70.48295565631028126, 0.000000000000000000 ) ) ;
#23112=AXIS2_PLACEMENT_3D ( 'NONE', #12612, #33369, #9865 ) ;
#23201=EDGE_CURVE ( 'NONE', #15184, #31380, #9372, .T. ) ;
#23206=EDGE_LOOP ( 'NONE', ( #29347, #12944, #1957, #10035 ) ) ;
#23213=EDGE_CURVE ( 'NONE', #30412, #19806, #14880, .T. ) ;
#23226=VERTEX_POINT ( 'NONE', #10601 ) ;
#23262=CIRCLE ( 'NONE', #23805, 32.63512777199724724 ) ;
#23277=CARTESIAN_POINT ( 'NONE',  ( 31.38736896855614944, -89.55944200217849982, 0.000000000000000000 ) ) ;
#23287=ORIENTED_EDGE ( 'NONE', *, *, #23296, .T. ) ;
#23296=EDGE_CURVE ( 'NONE', #6976, #3977, #8845, .T. ) ;
#23421=ORIENTED_EDGE ( 'NONE', *, *, #26046, .F. ) ;
#23461=DIRECTION ( 'NONE',  ( -1.224646799147353454E-16, 1.000000000000000000, -0.000000000000000000 ) ) ;
#23473=PRODUCT_CONTEXT ( 'NONE', #869, 'mechanical' ) ;
#23478=CARTESIAN_POINT ( 'NONE',  ( 10.69578794377714281, -43.58578643762690064, 2.566657756148792685E-15 ) ) ;
#23503=ORIENTED_EDGE ( 'NONE', *, *, #7258, .T. ) ;
#23582=ORIENTED_EDGE ( 'NONE', *, *, #17122, .T. ) ;
#23590=VERTEX_POINT ( 'NONE', #12099 ) ;
#23627=ORIENTED_EDGE ( 'NONE', *, *, #30730, .T. ) ;
#23656=CIRCLE ( 'NONE', #28025, 3.500000000000010214 ) ;
#23660=DIRECTION ( 'NONE',  ( 1.224646799147353454E-16, -1.000000000000000000, 0.000000000000000000 ) ) ;
#23666=AXIS2_PLACEMENT_3D ( 'NONE', #12866, #33969, #25089 ) ;
#23733=VECTOR ( 'NONE', #32634, 1000.000000000000000 ) ;
#23749=FACE_OUTER_BOUND ( 'NONE', #2940, .T. ) ;
#23786=LINE ( 'NONE', #31660, #14309 ) ;
#23794=DIRECTION ( 'NONE',  ( -1.224646799147353454E-16, 1.000000000000000000, -0.000000000000000000 ) ) ;
#23799=DIRECTION ( 'NONE',  ( -1.000000000000000000, 0.000000000000000000, 0.000000000000000000 ) ) ;
#23805=AXIS2_PLACEMENT_3D ( 'NONE', #28960, #13177, #18004 ) ;
#23818=CARTESIAN_POINT ( 'NONE',  ( 8.151180760100182884E-15, -89.55944200217849982, 0.000000000000000000 ) ) ;
#23839=ORIENTED_EDGE ( 'NONE', *, *, #29737, .F. ) ;
#23918=EDGE_LOOP ( 'NONE', ( #17238, #4276, #5597, #18256 ) ) ;
#23959=ADVANCED_FACE ( 'NONE', ( #25191 ), #30977, .T. ) ;
#23965=ORIENTED_EDGE ( 'NONE', *, *, #1063, .F. ) ;
#24009=ORIENTED_EDGE ( 'NONE', *, *, #3707, .T. ) ;
#24068=DIRECTION ( 'NONE',  ( 1.224646799147353454E-16, -1.000000000000000000, 0.000000000000000000 ) ) ;
#24071=ADVANCED_FACE ( 'NONE', ( #2367 ), #13454, .T. ) ;
#24101=DIRECTION ( 'NONE',  ( -1.000000000000000000, 0.000000000000000000, 0.000000000000000000 ) ) ;
#24131=ORIENTED_EDGE ( 'NONE', *, *, #22463, .F. ) ;
#24163=CARTESIAN_POINT ( 'NONE',  ( 12.11000150615022264, -45.00000000000001421, 0.000000000000000000 ) ) ;
#24173=AXIS2_PLACEMENT_3D ( 'NONE', #32018, #19000, #8682 ) ;
#24176=DIRECTION ( 'NONE',  ( -1.000000000000000000, -1.224646799147353454E-16, 0.000000000000000000 ) ) ;
#24180=CARTESIAN_POINT ( 'NONE',  ( 6.054684311146244891E-15, -72.44024934668307480, 0.000000000000000000 ) ) ;
#24199=CIRCLE ( 'NONE', #18185, 10.11607355459420177 ) ;
#24201=AXIS2_PLACEMENT_3D ( 'NONE', #30866, #265, #12342 ) ;
#24210=EDGE_CURVE ( 'NONE', #6224, #15184, #16109, .T. ) ;
#24229=DIRECTION ( 'NONE',  ( 1.224646799147353454E-16, -1.000000000000000000, 0.000000000000000000 ) ) ;
#24237=CARTESIAN_POINT ( 'NONE',  ( -12.11607355459419644, -70.99969134886156041, 0.000000000000000000 ) ) ;
#24263=CARTESIAN_POINT ( 'NONE',  ( -26.50000000000000355, -2.000000000000001332, 0.000000000000000000 ) ) ;
#24273=FACE_OUTER_BOUND ( 'NONE', #5259, .T. ) ;
#24294=ORIENTED_EDGE ( 'NONE', *, *, #5178, .T. ) ;
#24336=AXIS2_PLACEMENT_3D ( 'NONE', #17048, #6407, #3664 ) ;
#24340=EDGE_LOOP ( 'NONE', ( #26656, #10583, #25724, #12898 ) ) ;
#24355=COLOUR_RGB ( '', 0.66274510, 0.83137255, 0.94901961) ;
#24367=CARTESIAN_POINT ( 'NONE',  ( 4.222871413987100692E-15, -57.48236190979495319, 0.000000000000000000 ) ) ;
#24397=CIRCLE ( 'NONE', #5201, 26.50000000000000000 ) ;
#24416=ORIENTED_EDGE ( 'NONE', *, *, #5042, .T. ) ;
#24431=DIRECTION ( 'NONE',  ( -1.224646799147353454E-16, 1.000000000000000000, -0.000000000000000000 ) ) ;
#24459=CARTESIAN_POINT ( 'NONE',  ( 26.50000000000000000, -15.84529946162074943, 0.000000000000000000 ) ) ;
#24484=CARTESIAN_POINT ( 'NONE',  ( 4.349545668204547685E-15, -58.51673569255127205, 0.000000000000000000 ) ) ;
#24512=( LENGTH_UNIT ( ) NAMED_UNIT ( * ) SI_UNIT ( .MILLI., .METRE. ) );
#24513=VECTOR ( 'NONE', #229, 1000.000000000000114 ) ;
#24622=ADVANCED_FACE ( 'NONE', ( #1981 ), #7581, .T. ) ;
#24657=EDGE_CURVE ( 'NONE', #7743, #7355, #17330, .T. ) ;
#24661=ORIENTED_EDGE ( 'NONE', *, *, #10983, .T. ) ;
#24693=CARTESIAN_POINT ( 'NONE',  ( -24.49999999999999645, -23.00000000000000355, 0.000000000000000000 ) ) ;
#24718=DIRECTION ( 'NONE',  ( 0.000000000000000000, -0.000000000000000000, -1.000000000000000000 ) ) ;
#24826=VERTEX_POINT ( 'NONE', #31155 ) ;
#24842=SHAPE_REPRESENTATION_RELATIONSHIP ( 'NONE' , 'NONE' ,  #19696, #15260 ) ;
#24892=DIRECTION ( 'NONE',  ( -1.000000000000000000, 0.000000000000000000, 0.000000000000000000 ) ) ;
#24914=ORIENTED_EDGE ( 'NONE', *, *, #2379, .F. ) ;
#24971=FACE_OUTER_BOUND ( 'NONE', #20200, .T. ) ;
#24982=FACE_OUTER_BOUND ( 'NONE', #6600, .T. ) ;
#25022=FACE_OUTER_BOUND ( 'NONE', #21554, .T. ) ;
#25023=DIRECTION ( 'NONE',  ( -1.224646799147353454E-16, 1.000000000000000000, -0.000000000000000000 ) ) ;
#25082=ADVANCED_FACE ( 'NONE', ( #9523 ), #7289, .T. ) ;
#25086=CARTESIAN_POINT ( 'NONE',  ( -12.11000150615021553, -45.00000000000001421, 1.679354548928025724E-15 ) ) ;
#25089=DIRECTION ( 'NONE',  ( -1.000000000000000000, 0.000000000000000000, 0.000000000000000000 ) ) ;
#25094=AXIS2_PLACEMENT_3D ( 'NONE', #24484, #628, #958 ) ;
#25191=FACE_OUTER_BOUND ( 'NONE', #174, .T. ) ;
#25228=ADVANCED_FACE ( 'NONE', ( #24273 ), #10644, .F. ) ;
#25260=ORIENTED_EDGE ( 'NONE', *, *, #6275, .T. ) ;
#25292=AXIS2_PLACEMENT_3D ( 'NONE', #26386, #284, #10772 ) ;
#25293=AXIS2_PLACEMENT_3D ( 'NONE', #24180, #6141, #18868 ) ;
#25296=EDGE_CURVE ( 'NONE', #2254, #20157, #25976, .T. ) ;
#25298=ORIENTED_EDGE ( 'NONE', *, *, #8324, .T. ) ;
#25306=ORIENTED_EDGE ( 'NONE', *, *, #21821, .T. ) ;
#25337=CIRCLE ( 'NONE', #20354, 31.91025403784435710 ) ;
#25350=CARTESIAN_POINT ( 'NONE',  ( -12.11000150615021198, -45.00000000000000000, 0.000000000000000000 ) ) ;
#25367=CARTESIAN_POINT ( 'NONE',  ( -26.50000000000000000, -23.00000000000000355, 0.000000000000000000 ) ) ;
#25409=EDGE_LOOP ( 'NONE', ( #8370, #28590, #23965, #8372 ) ) ;
#25454=ORIENTED_EDGE ( 'NONE', *, *, #4609, .F. ) ;
#25504=CARTESIAN_POINT ( 'NONE',  ( 0.000000000000000000, -23.00000000000000000, 0.000000000000000000 ) ) ;
#25523=EDGE_CURVE ( 'NONE', #2254, #16950, #213, .T. ) ;
#25544=DIRECTION ( 'NONE',  ( 1.224646799147353454E-16, -1.000000000000000000, 0.000000000000000000 ) ) ;
#25545=DIRECTION ( 'NONE',  ( -1.000000000000000000, -1.239088197126291063E-16, 0.000000000000000000 ) ) ;
#25648=VERTEX_POINT ( 'NONE', #4508 ) ;
#25686=DIRECTION ( 'NONE',  ( -1.224646799147353454E-16, 1.000000000000000000, -0.000000000000000000 ) ) ;
#25712=DIRECTION ( 'NONE',  ( -1.000000000000000000, -1.122425893913996568E-16, 0.000000000000000000 ) ) ;
#25724=ORIENTED_EDGE ( 'NONE', *, *, #13072, .T. ) ;
#25733=DIRECTION ( 'NONE',  ( 1.224646799147353454E-16, -1.000000000000000000, 0.000000000000000000 ) ) ;
#25790=EDGE_LOOP ( 'NONE', ( #11412, #11451, #3487, #1257 ) ) ;
#25822=VECTOR ( 'NONE', #1000, 1000.000000000000000 ) ;
#25834=AXIS2_PLACEMENT_3D ( 'NONE', #23818, #26045, #33774 ) ;
#25855=TOROIDAL_SURFACE ( 'NONE', #23112, 11.45223628611452860, 4.000000000000014211 ) ;
#25894=AXIS2_PLACEMENT_3D ( 'NONE', #22128, #9071, #22798 ) ;
#25895=VECTOR ( 'NONE', #27398, 1000.000000000000000 ) ;
#25908=( NAMED_UNIT ( * ) SI_UNIT ( $, .STERADIAN. ) SOLID_ANGLE_UNIT ( ) );
#25954=DIRECTION ( 'NONE',  ( -1.224646799147353207E-16, -1.499759782661857882E-32, 1.000000000000000000 ) ) ;
#25959=LINE ( 'NONE', #10683, #33080 ) ;
#25969=UNCERTAINTY_MEASURE_WITH_UNIT (LENGTH_MEASURE( 1.000000000000000082E-05 ), #31394, 'distance_accuracy_value', 'NONE');
#25976=CIRCLE ( 'NONE', #24336, 1.500000000000008216 ) ;
#25978=DIRECTION ( 'NONE',  ( 1.000000000000000000, 1.416100796715761110E-16, 0.000000000000000000 ) ) ;
#25994=FACE_OUTER_BOUND ( 'NONE', #21510, .T. ) ;
#26045=DIRECTION ( 'NONE',  ( -1.224646799147353454E-16, 1.000000000000000000, -0.000000000000000000 ) ) ;
#26046=EDGE_CURVE ( 'NONE', #19445, #9464, #25959, .T. ) ;
#26051=CARTESIAN_POINT ( 'NONE',  ( 0.000000000000000000, -21.99999999999999645, 0.000000000000000000 ) ) ;
#26108=EDGE_LOOP ( 'NONE', ( #11330, #33157, #15187, #25454 ) ) ;
#26116=CARTESIAN_POINT ( 'NONE',  ( -7.347880794884122694E-16, -16.99999999999999645, 0.000000000000000000 ) ) ;
#26195=ORIENTED_EDGE ( 'NONE', *, *, #4418, .T. ) ;
#26230=DIRECTION ( 'NONE',  ( 1.000000000000000000, 0.000000000000000000, 0.000000000000000000 ) ) ;
#26386=CARTESIAN_POINT ( 'NONE',  ( 5.204170427930421283E-15, -70.99969134886156041, 0.000000000000000000 ) ) ;
#26412=ORIENTED_EDGE ( 'NONE', *, *, #3757, .T. ) ;
#26521=VECTOR ( 'NONE', #5838, 1000.000000000000114 ) ;
#26546=CARTESIAN_POINT ( 'NONE',  ( -4.936660134684515206E-16, -18.96891108675447768, 0.000000000000000000 ) ) ;
#26562=DIRECTION ( 'NONE',  ( 0.000000000000000000, -0.000000000000000000, -1.000000000000000000 ) ) ;
#26587=FACE_OUTER_BOUND ( 'NONE', #18990, .T. ) ;
#26598=FACE_OUTER_BOUND ( 'NONE', #25790, .T. ) ;
#26656=ORIENTED_EDGE ( 'NONE', *, *, #25523, .F. ) ;
#26672=AXIS2_PLACEMENT_3D ( 'NONE', #19092, #26964, #3465 ) ;
#26695=CONICAL_SURFACE ( 'NONE', #17358, 13.38432950954957157, 0.2613323016132363952 ) ;
#26748=ORIENTED_EDGE ( 'NONE', *, *, #6275, .F. ) ;
#26765=DIRECTION ( 'NONE',  ( -1.000000000000000000, -1.224646799147353454E-16, 0.000000000000000000 ) ) ;
#26770=UNCERTAINTY_MEASURE_WITH_UNIT (LENGTH_MEASURE( 1.000000000000000082E-05 ), #24512, 'distance_accuracy_value', 'NONE');
#26783=ORIENTED_EDGE ( 'NONE', *, *, #8324, .F. ) ;
#26829=DIRECTION ( 'NONE',  ( 0.000000000000000000, -0.000000000000000000, -1.000000000000000000 ) ) ;
#26930=CARTESIAN_POINT ( 'NONE',  ( 4.412827539393359662E-15, -59.03347138510255832, 0.000000000000000000 ) ) ;
#26940=DIRECTION ( 'NONE',  ( -1.224646799147353207E-16, -1.499759782661857882E-32, 1.000000000000000000 ) ) ;
#26950=FACE_OUTER_BOUND ( 'NONE', #10411, .T. ) ;
#26964=DIRECTION ( 'NONE',  ( -1.224646799147353454E-16, 1.000000000000000000, -0.000000000000000000 ) ) ;
#26985=ADVANCED_FACE ( 'NONE', ( #17250 ), #14385, .F. ) ;
#27000=DIRECTION ( 'NONE',  ( 1.224646799147353454E-16, -1.000000000000000000, 0.000000000000000000 ) ) ;
#27015=DIRECTION ( 'NONE',  ( -0.8660254037844363761, -0.5000000000000038858, 1.060575238724904326E-16 ) ) ;
#27017=AXIS2_PLACEMENT_3D ( 'NONE', #16100, #15927, #10934 ) ;
#27028=ORIENTED_EDGE ( 'NONE', *, *, #18187, .F. ) ;
#27039=EDGE_CURVE ( 'NONE', #23106, #12231, #31385, .T. ) ;
#27068=AXIS2_PLACEMENT_3D ( 'NONE', #30451, #30621, #17774 ) ;
#27135=CIRCLE ( 'NONE', #9593, 1.999999999999993117 ) ;
#27186=CARTESIAN_POINT ( 'NONE',  ( -13.38408793869266056, -57.48236190979495319, 1.639078045362666731E-15 ) ) ;
#27231=AXIS2_PLACEMENT_3D ( 'NONE', #30518, #27961, #33442 ) ;
#27274=EDGE_CURVE ( 'NONE', #16950, #2254, #7822, .T. ) ;
#27275=CARTESIAN_POINT ( 'NONE',  ( -12.11000150615021553, -45.00000000000001421, 1.483047458217649221E-15 ) ) ;
#27280=CIRCLE ( 'NONE', #30575, 3.500000000000010214 ) ;
#27281=DIRECTION ( 'NONE',  ( -1.000000000000000000, 0.000000000000000000, 0.000000000000000000 ) ) ;
#27321=DIRECTION ( 'NONE',  ( -1.224646799147353454E-16, 1.000000000000000000, -0.000000000000000000 ) ) ;
#27336=CARTESIAN_POINT ( 'NONE',  ( -15.31642273298460744, -59.03347138510255832, 0.000000000000000000 ) ) ;
#27398=DIRECTION ( 'NONE',  ( 0.8660254037844365982, -0.5000000000000036637, 0.000000000000000000 ) ) ;
#27418=CYLINDRICAL_SURFACE ( 'NONE', #11591, 26.50000000000000000 ) ;
#27431=DIRECTION ( 'NONE',  ( -1.000000000000000000, 0.000000000000000000, 0.000000000000000000 ) ) ;
#27449=ORIENTED_EDGE ( 'NONE', *, *, #19642, .F. ) ;
#27453=DIRECTION ( 'NONE',  ( -1.224646799147353454E-16, 1.000000000000000000, -0.000000000000000000 ) ) ;
#27460=DIRECTION ( 'NONE',  ( 0.000000000000000000, 0.000000000000000000, 1.000000000000000000 ) ) ;
#27464=EDGE_CURVE ( 'NONE', #28463, #30412, #29174, .T. ) ;
#27467=AXIS2_PLACEMENT_3D ( 'NONE', #29933, #14839, #6437 ) ;
#27495=VERTEX_POINT ( 'NONE', #24263 ) ;
#27529=DIRECTION ( 'NONE',  ( -1.000000000000000000, 0.000000000000000000, 0.000000000000000000 ) ) ;
#27561=CARTESIAN_POINT ( 'NONE',  ( -31.91025403784435710, -18.96891108675448123, 0.000000000000000000 ) ) ;
#27603=FACE_OUTER_BOUND ( 'NONE', #30785, .T. ) ;
#27605=CONICAL_SURFACE ( 'NONE', #2408, 24.49999999999999645, 1.047197551196593412 ) ;
#27641=ORIENTED_EDGE ( 'NONE', *, *, #23201, .F. ) ;
#27674=DIRECTION ( 'NONE',  ( -1.224646799147353454E-16, 1.000000000000000000, -0.000000000000000000 ) ) ;
#27682=ORIENTED_EDGE ( 'NONE', *, *, #4526, .T. ) ;
#27703=EDGE_CURVE ( 'NONE', #7457, #7617, #6724, .T. ) ;
#27710=CARTESIAN_POINT ( 'NONE',  ( 8.305033359366087120E-16, -29.78157438140398483, 0.000000000000000000 ) ) ;
#27744=EDGE_CURVE ( 'NONE', #24826, #6976, #10573, .T. ) ;
#27762=CIRCLE ( 'NONE', #16274, 15.31642273298461276 ) ;
#27766=EDGE_CURVE ( 'NONE', #7617, #11830, #29723, .T. ) ;
#27772=CARTESIAN_POINT ( 'NONE',  ( -30.91025403784432513, -20.70096189432334910, 3.785414366827760066E-15 ) ) ;
#27788=VECTOR ( 'NONE', #27015, 999.9999999999998863 ) ;
#27790=CARTESIAN_POINT ( 'NONE',  ( -26.50000000000000000, -15.84529946162075653, 3.576596532241492659E-15 ) ) ;
#27813=ORIENTED_EDGE ( 'NONE', *, *, #16089, .T. ) ;
#27822=VECTOR ( 'NONE', #32306, 1000.000000000000114 ) ;
#27842=CARTESIAN_POINT ( 'NONE',  ( 8.327598234202002696E-15, -91.00000000000000000, 0.000000000000000000 ) ) ;
#27878=VERTEX_POINT ( 'NONE', #25086 ) ;
#27889=CARTESIAN_POINT ( 'NONE',  ( 2.521031746877078694E-15, -43.58578643762690064, 0.000000000000000000 ) ) ;
#27961=DIRECTION ( 'NONE',  ( 1.224646799147353454E-16, -1.000000000000000000, 0.000000000000000000 ) ) ;
#28008=CIRCLE ( 'NONE', #1136, 12.11000150615021909 ) ;
#28025=AXIS2_PLACEMENT_3D ( 'NONE', #10340, #2949, #13421 ) ;
#28037=AXIS2_PLACEMENT_3D ( 'NONE', #27842, #143, #28476 ) ;
#28040=ADVANCED_FACE ( 'NONE', ( #2262 ), #17136, .F. ) ;
#28085=EDGE_CURVE ( 'NONE', #23226, #7457, #4536, .T. ) ;
#28090=DIRECTION ( 'NONE',  ( 1.000000000000000000, 0.000000000000000000, 1.224646799147352714E-16 ) ) ;
#28103=AXIS2_PLACEMENT_3D ( 'NONE', #18784, #26829, #8631 ) ;
#28135=EDGE_CURVE ( 'NONE', #33921, #19806, #8911, .T. ) ;
#28174=AXIS2_PLACEMENT_3D ( 'NONE', #33981, #12707, #21122 ) ;
#28191=CARTESIAN_POINT ( 'NONE',  ( -10.69578794377713926, -43.58578643762690064, 0.000000000000000000 ) ) ;
#28228=CARTESIAN_POINT ( 'NONE',  ( 15.31593959127081739, -56.96472381958990638, 1.875691223536068310E-15 ) ) ;
#28241=CARTESIAN_POINT ( 'NONE',  ( 0.000000000000000000, -21.99999999999999645, 0.000000000000000000 ) ) ;
#28244=( GEOMETRIC_REPRESENTATION_CONTEXT ( 3 ) GLOBAL_UNCERTAINTY_ASSIGNED_CONTEXT ( ( #31115 ) ) GLOBAL_UNIT_ASSIGNED_CONTEXT ( ( #33213, #22585, #14529 ) ) REPRESENTATION_CONTEXT ( 'NONE', 'WORKASPACE' ) );
#28279=AXIS2_PLACEMENT_3D ( 'NONE', #22324, #24718, #1195 ) ;
#28351=DIRECTION ( 'NONE',  ( -1.224646799147353454E-16, 1.000000000000000000, -0.000000000000000000 ) ) ;
#28388=ORIENTED_EDGE ( 'NONE', *, *, #12946, .T. ) ;
#28463=VERTEX_POINT ( 'NONE', #1612 ) ;
#28476=DIRECTION ( 'NONE',  ( -1.000000000000000000, 0.000000000000000000, 0.000000000000000000 ) ) ;
#28503=EDGE_LOOP ( 'NONE', ( #29714, #11826 ) ) ;
#28529=VERTEX_POINT ( 'NONE', #29767 ) ;
#28590=ORIENTED_EDGE ( 'NONE', *, *, #18312, .T. ) ;
#28617=DIRECTION ( 'NONE',  ( -1.000000000000000000, -1.224646799147353454E-16, 0.000000000000000000 ) ) ;
#28661=CONICAL_SURFACE ( 'NONE', #1797, 12.11000150615021909, 0.2617993877991545149 ) ;
#28678=ORIENTED_EDGE ( 'NONE', *, *, #3707, .F. ) ;
#28689=CARTESIAN_POINT ( 'NONE',  ( 10.11000150615022619, -45.00000000000000000, 1.238118098388178925E-15 ) ) ;
#28690=CIRCLE ( 'NONE', #2383, 15.31642273298461276 ) ;
#28758=STYLED_ITEM ( 'NONE', ( #22761 ), #33133 ) ;
#28813=CIRCLE ( 'NONE', #7998, 30.91025403784432868 ) ;
#28815=CARTESIAN_POINT ( 'NONE',  ( 15.31642273298461632, -59.03347138510255832, 1.875720807433735970E-15 ) ) ;
#28853=AXIS2_PLACEMENT_3D ( 'NONE', #28241, #20013, #19835 ) ;
#28953=CARTESIAN_POINT ( 'NONE',  ( 5.204170427930421283E-15, -70.99969134886156041, 0.000000000000000000 ) ) ;
#28960=CARTESIAN_POINT ( 'NONE',  ( 1.806199397676865774E-16, -24.47487373415291145, 0.000000000000000000 ) ) ;
#28972=ORIENTED_EDGE ( 'NONE', *, *, #12161, .F. ) ;
#29108=AXIS2_PLACEMENT_3D ( 'NONE', #3083, #10803, #21444 ) ;
#29112=CARTESIAN_POINT ( 'NONE',  ( -4.936660134684515206E-16, -18.96891108675447768, 0.000000000000000000 ) ) ;
#29174=CIRCLE ( 'NONE', #28103, 1.999999999999993117 ) ;
#29179=ORIENTED_EDGE ( 'NONE', *, *, #5042, .F. ) ;
#29250=CIRCLE ( 'NONE', #17183, 2.000000000000013767 ) ;
#29257=VERTEX_POINT ( 'NONE', #2789 ) ;
#29271=CONICAL_SURFACE ( 'NONE', #6245, 10.17814985357208890, 0.2617993877991527385 ) ;
#29273=ADVANCED_FACE ( 'NONE', ( #18755 ), #29750, .F. ) ;
#29319=FILL_AREA_STYLE ('',( #18204 ) ) ;
#29332=AXIS2_PLACEMENT_3D ( 'NONE', #12323, #11978, #20577 ) ;
#29347=ORIENTED_EDGE ( 'NONE', *, *, #30730, .F. ) ;
#29352=DIRECTION ( 'NONE',  ( -1.000000000000000000, -1.416100796715760863E-16, 0.000000000000000000 ) ) ;
#29375=AXIS2_PLACEMENT_3D ( 'NONE', #7935, #15332, #4679 ) ;
#29557=LINE ( 'NONE', #27336, #27822 ) ;
#29604=DIRECTION ( 'NONE',  ( -1.000000000000000000, -1.087251435804610394E-16, 0.000000000000000000 ) ) ;
#29616=DIRECTION ( 'NONE',  ( -1.000000000000000000, 0.000000000000000000, 0.000000000000000000 ) ) ;
#29656=AXIS2_PLACEMENT_3D ( 'NONE', #110, #10431, #7680 ) ;
#29714=ORIENTED_EDGE ( 'NONE', *, *, #4526, .F. ) ;
#29723=CIRCLE ( 'NONE', #14953, 24.49999999999999645 ) ;
#29737=EDGE_CURVE ( 'NONE', #4339, #21971, #2357, .T. ) ;
#29750=CONICAL_SURFACE ( 'NONE', #12219, 10.72870458603808075, 0.8042044335707554392 ) ;
#29767=CARTESIAN_POINT ( 'NONE',  ( 13.38408793869266766, -57.48236190979495319, 0.000000000000000000 ) ) ;
#29772=CIRCLE ( 'NONE', #8079, 12.11607355459420354 ) ;
#29778=ADVANCED_FACE ( 'NONE', ( #20553 ), #8938, .T. ) ;
#29841=EDGE_CURVE ( 'NONE', #24826, #13703, #20472, .T. ) ;
#29863=DIRECTION ( 'NONE',  ( -1.224646799147353454E-16, 1.000000000000000000, -0.000000000000000000 ) ) ;
#29896=DIRECTION ( 'NONE',  ( 1.000000000000000000, 0.000000000000000000, 1.224646799147353454E-16 ) ) ;
#29933=CARTESIAN_POINT ( 'NONE',  ( 3.469446951953614189E-15, -57.99999999999999289, 0.000000000000000000 ) ) ;
#30012=AXIS2_PLACEMENT_3D ( 'NONE', #8358, #11280, #29616 ) ;
#30162=DIRECTION ( 'NONE',  ( -1.224646799147353454E-16, 1.000000000000000000, -0.000000000000000000 ) ) ;
#30182=CONICAL_SURFACE ( 'NONE', #16520, 12.11607355459420354, 0.8042044335707554392 ) ;
#30221=ORIENTED_EDGE ( 'NONE', *, *, #17841, .T. ) ;
#30266=ORIENTED_EDGE ( 'NONE', *, *, #12946, .F. ) ;
#30392=EDGE_CURVE ( 'NONE', #7411, #28529, #29250, .T. ) ;
#30402=CIRCLE ( 'NONE', #18926, 31.38736896855613523 ) ;
#30404=DIRECTION ( 'NONE',  ( 1.000000000000000000, 0.000000000000000000, 1.224646799147353454E-16 ) ) ;
#30412=VERTEX_POINT ( 'NONE', #8737 ) ;
#30437=EDGE_CURVE ( 'NONE', #17976, #28529, #18856, .T. ) ;
#30451=CARTESIAN_POINT ( 'NONE',  ( 0.000000000000000000, -23.00000000000000000, 0.000000000000000000 ) ) ;
#30466=CARTESIAN_POINT ( 'NONE',  ( 10.17814985357209245, -45.51763809020504681, 1.246463863941915697E-15 ) ) ;
#30500=CARTESIAN_POINT ( 'NONE',  ( 4.349545668204547685E-15, -58.51673569255127205, 0.000000000000000000 ) ) ;
#30518=CARTESIAN_POINT ( 'NONE',  ( 5.878266837044421923E-15, -70.99969134886156041, 0.000000000000000000 ) ) ;
#30538=DIRECTION ( 'NONE',  ( -1.000000000000000000, -1.224646799147353454E-16, 0.000000000000000000 ) ) ;
#30542=EDGE_CURVE ( 'NONE', #25648, #20029, #28690, .T. ) ;
#30565=ORIENTED_EDGE ( 'NONE', *, *, #4418, .F. ) ;
#30569=DIRECTION ( 'NONE',  ( 0.000000000000000000, -0.000000000000000000, -1.000000000000000000 ) ) ;
#30575=AXIS2_PLACEMENT_3D ( 'NONE', #21694, #32638, #29896 ) ;
#30592=FACE_OUTER_BOUND ( 'NONE', #15825, .T. ) ;
#30621=DIRECTION ( 'NONE',  ( -1.224646799147353454E-16, 1.000000000000000000, -0.000000000000000000 ) ) ;
#30630=DIRECTION ( 'NONE',  ( -1.224646799147353454E-16, 1.000000000000000000, -0.000000000000000000 ) ) ;
#30730=EDGE_CURVE ( 'NONE', #4339, #15184, #32575, .T. ) ;
#30776=DIRECTION ( 'NONE',  ( 1.224646799147353454E-16, -1.000000000000000000, 0.000000000000000000 ) ) ;
#30785=EDGE_LOOP ( 'NONE', ( #19273, #4356, #15439, #5000 ) ) ;
#30832=CIRCLE ( 'NONE', #676, 24.49999999999999645 ) ;
#30866=CARTESIAN_POINT ( 'NONE',  ( 2.694222958124179176E-15, -45.00000000000001421, 0.000000000000000000 ) ) ;
#30885=CARTESIAN_POINT ( 'NONE',  ( -32.63512777199724724, -24.47487373415291501, 0.000000000000000000 ) ) ;
#30977=CONICAL_SURFACE ( 'NONE', #29332, 30.00000000000000711, 0.7665918932241471140 ) ;
#31090=ORIENTED_EDGE ( 'NONE', *, *, #13215, .F. ) ;
#31115=UNCERTAINTY_MEASURE_WITH_UNIT (LENGTH_MEASURE( 1.000000000000000082E-05 ), #33213, 'distance_accuracy_value', 'NONE');
#31155=CARTESIAN_POINT ( 'NONE',  ( -10.18398033115917123, -70.48295565631028126, 0.000000000000000000 ) ) ;
#31169=ORIENTED_EDGE ( 'NONE', *, *, #18312, .F. ) ;
#31258=CARTESIAN_POINT ( 'NONE',  ( 3.469446951953614189E-15, -57.99999999999999289, 0.000000000000000000 ) ) ;
#31267=ADVANCED_FACE ( 'NONE', ( #2720 ), #13365, .F. ) ;
#31290=ORIENTED_EDGE ( 'NONE', *, *, #7894, .T. ) ;
#31292=DIRECTION ( 'NONE',  ( 0.6936844842780659492, 0.7202789989107510893, 8.495184832893160525E-17 ) ) ;
#31354=CARTESIAN_POINT ( 'NONE',  ( -31.38736896855613523, -89.55944200217849982, 3.843844094099923719E-15 ) ) ;
#31380=VERTEX_POINT ( 'NONE', #23277 ) ;
#31385=CIRCLE ( 'NONE', #12752, 10.69578794377714104 ) ;
#31394=( LENGTH_UNIT ( ) NAMED_UNIT ( * ) SI_UNIT ( .MILLI., .METRE. ) );
#31422=ORIENTED_EDGE ( 'NONE', *, *, #14830, .F. ) ;
#31462=ORIENTED_EDGE ( 'NONE', *, *, #17122, .F. ) ;
#31524=DIRECTION ( 'NONE',  ( -1.224646799147353454E-16, 1.000000000000000000, -0.000000000000000000 ) ) ;
#31553=AXIS2_PLACEMENT_3D ( 'NONE', #20265, #10135, #30538 ) ;
#31569=DIRECTION ( 'NONE',  ( -1.000000000000000000, 0.000000000000000000, 0.000000000000000000 ) ) ;
#31627=DIRECTION ( 'NONE',  ( 0.8660254037844371533, -0.5000000000000026645, 0.000000000000000000 ) ) ;
#31630=ORIENTED_EDGE ( 'NONE', *, *, #27039, .T. ) ;
#31637=TOROIDAL_SURFACE ( 'NONE', #3165, 12.11000150615021553, 1.999999999999992228 ) ;
#31660=CARTESIAN_POINT ( 'NONE',  ( 13.38432950954957690, -58.51673569255127205, 1.639107629260334588E-15 ) ) ;
#31771=DIRECTION ( 'NONE',  ( 1.000000000000000000, 0.000000000000000000, 0.000000000000000000 ) ) ;
#31790=ADVANCED_FACE ( 'NONE', ( #19306 ), #21619, .T. ) ;
#31838=LINE ( 'NONE', #32005, #3375 ) ;
#31912=VECTOR ( 'NONE', #32658, 1000.000000000000000 ) ;
#31951=VECTOR ( 'NONE', #5285, 999.9999999999998863 ) ;
#31973=CARTESIAN_POINT ( 'NONE',  ( -30.16025403784430736, -22.00000000000000000, 0.000000000000000000 ) ) ;
#32005=CARTESIAN_POINT ( 'NONE',  ( -10.72870458603807542, -72.44024934668307480, 1.313887373028906602E-15 ) ) ;
#32018=CARTESIAN_POINT ( 'NONE',  ( 1.806199397676865774E-16, -24.47487373415291145, 0.000000000000000000 ) ) ;
#32058=( NAMED_UNIT ( * ) SI_UNIT ( $, .STERADIAN. ) SOLID_ANGLE_UNIT ( ) );
#32083=EDGE_LOOP ( 'NONE', ( #18270, #9124, #4682, #2387 ) ) ;
#32110=DIRECTION ( 'NONE',  ( -1.000000000000000000, 0.000000000000000000, 0.000000000000000000 ) ) ;
#32135=ORIENTED_EDGE ( 'NONE', *, *, #30437, .F. ) ;
#32147=DIRECTION ( 'NONE',  ( 1.000000000000000000, 1.416100796715761110E-16, 0.000000000000000000 ) ) ;
#32148=VECTOR ( 'NONE', #31292, 999.9999999999998863 ) ;
#32171=CARTESIAN_POINT ( 'NONE',  ( 26.50000000000000000, -22.99999999999999645, 3.245314017740485765E-15 ) ) ;
#32222=EDGE_CURVE ( 'NONE', #27878, #1088, #14239, .T. ) ;
#32306=DIRECTION ( 'NONE',  ( -0.2583678462756402450, 0.9660466117175128264, 0.000000000000000000 ) ) ;
#32312=CARTESIAN_POINT ( 'NONE',  ( -24.50000000000000000, -2.000000000000001332, 0.000000000000000000 ) ) ;
#32348=EDGE_CURVE ( 'NONE', #31380, #15184, #30402, .T. ) ;
#32419=ORIENTED_EDGE ( 'NONE', *, *, #33984, .T. ) ;
#32435=CARTESIAN_POINT ( 'NONE',  ( -2.815509657234710744E-16, -20.70096189432334555, 0.000000000000000000 ) ) ;
#32574=DIRECTION ( 'NONE',  ( -1.224646799147353454E-16, 1.000000000000000000, -0.000000000000000000 ) ) ;
#32575=LINE ( 'NONE', #16316, #26521 ) ;
#32586=ORIENTED_EDGE ( 'NONE', *, *, #22144, .T. ) ;
#32601=AXIS2_PLACEMENT_3D ( 'NONE', #26051, #10607, #12840 ) ;
#32620=AXIS2_PLACEMENT_3D ( 'NONE', #17689, #22483, #22828 ) ;
#32622=EDGE_CURVE ( 'NONE', #27495, #23590, #24397, .T. ) ;
#32632=ORIENTED_EDGE ( 'NONE', *, *, #6845, .F. ) ;
#32634=DIRECTION ( 'NONE',  ( -1.224646799147353454E-16, 1.000000000000000000, -0.000000000000000000 ) ) ;
#32638=DIRECTION ( 'NONE',  ( -1.224646799147353207E-16, -1.499759782661857882E-32, 1.000000000000000000 ) ) ;
#32646=DIRECTION ( 'NONE',  ( -1.000000000000000000, -1.111257322145974683E-16, 0.000000000000000000 ) ) ;
#32658=DIRECTION ( 'NONE',  ( 0.7071067811865465735, 0.7071067811865484609, 8.659560562354922997E-17 ) ) ;
#32696=CYLINDRICAL_SURFACE ( 'NONE', #16223, 24.49999999999999645 ) ;
#32751=VECTOR ( 'NONE', #1503, 1000.000000000000000 ) ;
#32881=DIRECTION ( 'NONE',  ( -1.224646799147353454E-16, 1.000000000000000000, -0.000000000000000000 ) ) ;
#32901=CARTESIAN_POINT ( 'NONE',  ( 3.469446951953614189E-15, -45.00000000000000000, 0.000000000000000000 ) ) ;
#32933=AXIS2_PLACEMENT_3D ( 'NONE', #17906, #22869, #30404 ) ;
#32957=AXIS2_PLACEMENT_3D ( 'NONE', #27889, #20342, #4373 ) ;
#33001=AXIS2_PLACEMENT_3D ( 'NONE', #22511, #30569, #9466 ) ;
#33080=VECTOR ( 'NONE', #2453, 1000.000000000000114 ) ;
#33091=CARTESIAN_POINT ( 'NONE',  ( 24.50000000000000000, -29.78157438140398128, 3.000384657911015469E-15 ) ) ;
#33133=MANIFOLD_SOLID_BREP ( 'Revolve-Thin1', #210 ) ;
#33157=ORIENTED_EDGE ( 'NONE', *, *, #5600, .T. ) ;
#33203=CARTESIAN_POINT ( 'NONE',  ( -8.761981113183991350E-16, -15.84529946162075298, 0.000000000000000000 ) ) ;
#33213=( LENGTH_UNIT ( ) NAMED_UNIT ( * ) SI_UNIT ( .MILLI., .METRE. ) );
#33248=CIRCLE ( 'NONE', #17364, 15.31593959127081384 ) ;
#33250=LINE ( 'NONE', #25367, #32751 ) ;
#33304=AXIS2_PLACEMENT_3D ( 'NONE', #16111, #26562, #464 ) ;
#33327=DIRECTION ( 'NONE',  ( 1.000000000000000000, 0.000000000000000000, 1.224646799147353454E-16 ) ) ;
#33369=DIRECTION ( 'NONE',  ( -1.224646799147353454E-16, 1.000000000000000000, -0.000000000000000000 ) ) ;
#33442=DIRECTION ( 'NONE',  ( 1.000000000000000000, 0.000000000000000000, 0.000000000000000000 ) ) ;
#33473=LINE ( 'NONE', #8990, #31912 ) ;
#33581=AXIS2_PLACEMENT_3D ( 'NONE', #13217, #21126, #31569 ) ;
#33593=EDGE_CURVE ( 'NONE', #23106, #33921, #27135, .T. ) ;
#33613=EDGE_LOOP ( 'NONE', ( #28678, #10372, #2898, #21386 ) ) ;
#33662=AXIS2_PLACEMENT_3D ( 'NONE', #16201, #21182, #3150 ) ;
#33774=DIRECTION ( 'NONE',  ( -1.000000000000000000, 0.000000000000000000, 0.000000000000000000 ) ) ;
#33921=VERTEX_POINT ( 'NONE', #28689 ) ;
#33923=DIRECTION ( 'NONE',  ( -1.000000000000000000, 0.000000000000000000, 0.000000000000000000 ) ) ;
#33969=DIRECTION ( 'NONE',  ( -1.224646799147353454E-16, 1.000000000000000000, -0.000000000000000000 ) ) ;
#33981=CARTESIAN_POINT ( 'NONE',  ( 3.469446951953614189E-15, -57.99999999999999289, 0.000000000000000000 ) ) ;
#33984=EDGE_CURVE ( 'NONE', #7355, #5385, #15835, .T. ) ;
ENDSEC;
END-ISO-10303-21;
